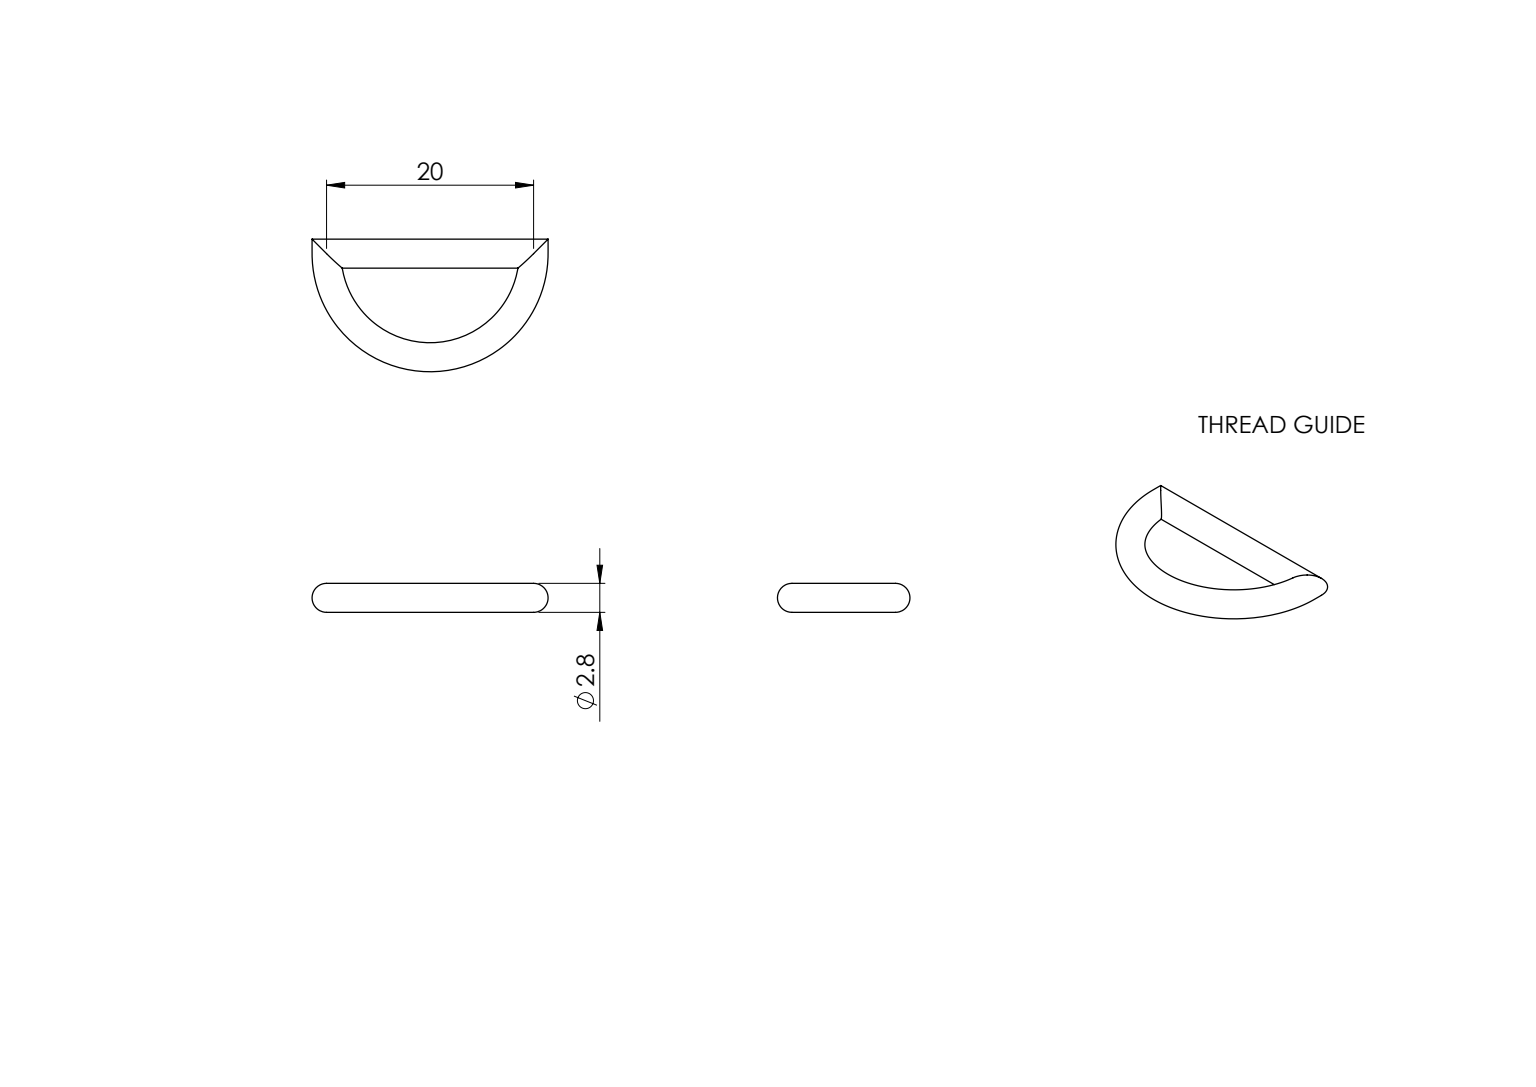
ISO-10303-21;
HEADER;
FILE_DESCRIPTION (('STEP AP214'),
    '1' );
FILE_NAME ('thread guide.step',
    '2026-10-25T11:00:22',
    ( '' ),
    ( '' ),
    'SwSTEP 2.0',
    'SolidWorks 2026',
    '' );
FILE_SCHEMA (( 'AUTOMOTIVE_DESIGN' ));
ENDSEC;

DATA;
#1=CARTESIAN_POINT ( 'NONE',  ( -6.877134118866000456, -50.00000000000000000, 5.285102517561346858 ) ) ;
#2=CARTESIAN_POINT ( 'NONE',  ( 11.39999999999999680, -52.79999999999999716, -0.5466666666666269991 ) ) ;
#3=ORIENTED_EDGE ( 'NONE', *, *, #2173, .T. ) ;
#9=( BOUNDED_SURFACE ( )  B_SPLINE_SURFACE ( 3, 3, ( 
 ( #2907, #429, #2418, #2187, #1154, #2219, #2974, #1713, #2728, #2169, #3178, #2938, #2958, #2662, #1219, #461, #1468, #698, #2482, #1435, #1899, #2449, #446, #1450, #649, #2462, #2236, #1651, #919, #1916, #663, #189, #680, #1664, #2679, #1419, #2432, #1171 ),
 ( #1682, #1596, #593, #2589, #838, #2249, #321, #302, #69, #2812, #1788, #1838, #1822, #2342, #3004, #817, #221, #2743, #3255, #1078, #1549, #337, #2094, #1730, #1292, #477, #787, #726, #801, #2001, #1486, #2308, #35, #2797, #984, #1343, #1045, #2610 ),
 ( #1233, #3101, #969, #2498, #1313, #2829, #1806, #2077, #1985, #559, #540, #2056, #2554, #1328, #2847, #2358, #2989, #285, #3065, #1561, #2324, #2567, #52, #1064, #3081, #575, #1578, #884, #87, #2898, #388, #899, #2112, #1910, #2672, #2930, #2396, #671 ),
 ( #372, #1672, #2689, #855, #150, #2916, #657, #3139, #1613, #1892, #2377, #3120, #2426, #2628, #912, #1163, #1925, #1131, #122, #2145, #1855, #3152, #2131, #1097, #2866, #2181, #1412, #643, #872, #608, #3185, #1629, #1644, #1873, #420, #2411, #1428, #1658 ),
 ( #355, #3169, #107, #2882, #627, #1362, #1116, #402, #2642, #1381, #2658, #1395, #134, #1145, #2162, #438, #2194, #736, #994, #1194, #961, #487, #1496, #2504, #1179, #2257, #705, #3234, #2210, #2763, #1476, #228, #1993, #453, #2492, #1444, #214, #1227 ),
 ( #1241, #167, #2751, #2011, #3265, #2456, #720, #499, #182, #2736, #3213, #3199, #1741, #3013, #943, #1978, #752, #1753, #2441, #2243, #1691, #927, #1961, #1941, #2967, #2949, #688, #2707, #2722, #1705, #1458, #2474, #2228, #198, #1210, #2981, #1722, #470 ),
 ( #3249, #975, #2998, #813, #765, #315, #1507, #1256, #797, #1307, #2303, #2564, #2519, #31, #1, #1784, #1768, #1817, #2823, #571, #1574, #1011, #2026, #1544, #2808, #2271, #830, #1323, #2582, #1801, #2338, #1039, #246, #2052, #554, #2319, #3026, #48 ) ),
 .UNSPECIFIED., .T., .F., .F. ) 
 B_SPLINE_SURFACE_WITH_KNOTS ( ( 4, 3, 4 ),
 ( 4, 2, 2, 2, 2, 2, 2, 2, 2, 2, 2, 2, 2, 2, 2, 2, 2, 2, 4 ),
 ( 0.000000000000000000, 0.5000000000000000000, 1.000000000000000000 ),
 ( -0.05205660780589810299, -0.02602830390294905150, 0.000000000000000000, 0.01562500000000000000, 0.03125000000000000000, 0.06250000000000000000, 0.1250000000000000000, 0.2500000000000000000, 0.3750000000000000000, 0.5000000000000000000, 0.6250000000000000000, 0.7500000000000000000, 0.8750000000000000000, 0.9375000000000000000, 0.9687500000000000000, 0.9843750000000000000, 1.000000000000000000, 1.026028303902949190, 1.052056607805898381 ),
 .UNSPECIFIED. ) 
 GEOMETRIC_REPRESENTATION_ITEM ( )  RATIONAL_B_SPLINE_SURFACE ( (
 ( 1.000000000000000000, 1.000000000000000000, 1.000000000000000000, 1.000000000000000000, 1.000000000000000000, 1.000000000000000000, 1.000000000000000000, 1.000000000000000000, 1.000000000000000000, 1.000000000000000000, 1.000000000000000000, 1.000000000000000000, 1.000000000000000000, 1.000000000000000000, 1.000000000000000000, 1.000000000000000000, 1.000000000000000000, 1.000000000000000000, 1.000000000000000000, 1.000000000000000000, 1.000000000000000000, 1.000000000000000000, 1.000000000000000000, 1.000000000000000000, 1.000000000000000000, 1.000000000000000000, 1.000000000000000000, 1.000000000000000000, 1.000000000000000000, 1.000000000000000000, 1.000000000000000000, 1.000000000000000000, 1.000000000000000000, 1.000000000000000000, 1.000000000000000000, 1.000000000000000000, 1.000000000000000000, 1.000000000000000000),
 ( 0.3333333333333333703, 0.3333333333333333703, 0.3333333333333333703, 0.3333333333333333703, 0.3333333333333333703, 0.3333333333333333703, 0.3333333333333333703, 0.3333333333333333703, 0.3333333333333333703, 0.3333333333333333703, 0.3333333333333333703, 0.3333333333333333703, 0.3333333333333333703, 0.3333333333333333703, 0.3333333333333333703, 0.3333333333333333703, 0.3333333333333333703, 0.3333333333333333703, 0.3333333333333333703, 0.3333333333333333703, 0.3333333333333333703, 0.3333333333333333703, 0.3333333333333333703, 0.3333333333333333703, 0.3333333333333333703, 0.3333333333333333703, 0.3333333333333333703, 0.3333333333333333703, 0.3333333333333333703, 0.3333333333333333703, 0.3333333333333333703, 0.3333333333333333703, 0.3333333333333333703, 0.3333333333333333703, 0.3333333333333333703, 0.3333333333333333703, 0.3333333333333333703, 0.3333333333333333703),
 ( 0.3333333333333333703, 0.3333333333333333703, 0.3333333333333333703, 0.3333333333333333703, 0.3333333333333333703, 0.3333333333333333703, 0.3333333333333333703, 0.3333333333333333703, 0.3333333333333333703, 0.3333333333333333703, 0.3333333333333333703, 0.3333333333333333703, 0.3333333333333333703, 0.3333333333333333703, 0.3333333333333333703, 0.3333333333333333703, 0.3333333333333333703, 0.3333333333333333703, 0.3333333333333333703, 0.3333333333333333703, 0.3333333333333333703, 0.3333333333333333703, 0.3333333333333333703, 0.3333333333333333703, 0.3333333333333333703, 0.3333333333333333703, 0.3333333333333333703, 0.3333333333333333703, 0.3333333333333333703, 0.3333333333333333703, 0.3333333333333333703, 0.3333333333333333703, 0.3333333333333333703, 0.3333333333333333703, 0.3333333333333333703, 0.3333333333333333703, 0.3333333333333333703, 0.3333333333333333703),
 ( 1.000000000000000000, 1.000000000000000000, 1.000000000000000000, 1.000000000000000000, 1.000000000000000000, 1.000000000000000000, 1.000000000000000000, 1.000000000000000000, 1.000000000000000000, 1.000000000000000000, 1.000000000000000000, 1.000000000000000000, 1.000000000000000000, 1.000000000000000000, 1.000000000000000000, 1.000000000000000000, 1.000000000000000000, 1.000000000000000000, 1.000000000000000000, 1.000000000000000000, 1.000000000000000000, 1.000000000000000000, 1.000000000000000000, 1.000000000000000000, 1.000000000000000000, 1.000000000000000000, 1.000000000000000000, 1.000000000000000000, 1.000000000000000000, 1.000000000000000000, 1.000000000000000000, 1.000000000000000000, 1.000000000000000000, 1.000000000000000000, 1.000000000000000000, 1.000000000000000000, 1.000000000000000000, 1.000000000000000000),
 ( 0.3333333333333333703, 0.3333333333333333703, 0.3333333333333333703, 0.3333333333333333703, 0.3333333333333333703, 0.3333333333333333703, 0.3333333333333333703, 0.3333333333333333703, 0.3333333333333333703, 0.3333333333333333703, 0.3333333333333333703, 0.3333333333333333703, 0.3333333333333333703, 0.3333333333333333703, 0.3333333333333333703, 0.3333333333333333703, 0.3333333333333333703, 0.3333333333333333703, 0.3333333333333333703, 0.3333333333333333703, 0.3333333333333333703, 0.3333333333333333703, 0.3333333333333333703, 0.3333333333333333703, 0.3333333333333333703, 0.3333333333333333703, 0.3333333333333333703, 0.3333333333333333703, 0.3333333333333333703, 0.3333333333333333703, 0.3333333333333333703, 0.3333333333333333703, 0.3333333333333333703, 0.3333333333333333703, 0.3333333333333333703, 0.3333333333333333703, 0.3333333333333333703, 0.3333333333333333703),
 ( 0.3333333333333333703, 0.3333333333333333703, 0.3333333333333333703, 0.3333333333333333703, 0.3333333333333333703, 0.3333333333333333703, 0.3333333333333333703, 0.3333333333333333703, 0.3333333333333333703, 0.3333333333333333703, 0.3333333333333333703, 0.3333333333333333703, 0.3333333333333333703, 0.3333333333333333703, 0.3333333333333333703, 0.3333333333333333703, 0.3333333333333333703, 0.3333333333333333703, 0.3333333333333333703, 0.3333333333333333703, 0.3333333333333333703, 0.3333333333333333703, 0.3333333333333333703, 0.3333333333333333703, 0.3333333333333333703, 0.3333333333333333703, 0.3333333333333333703, 0.3333333333333333703, 0.3333333333333333703, 0.3333333333333333703, 0.3333333333333333703, 0.3333333333333333703, 0.3333333333333333703, 0.3333333333333333703, 0.3333333333333333703, 0.3333333333333333703, 0.3333333333333333703, 0.3333333333333333703),
 ( 1.000000000000000000, 1.000000000000000000, 1.000000000000000000, 1.000000000000000000, 1.000000000000000000, 1.000000000000000000, 1.000000000000000000, 1.000000000000000000, 1.000000000000000000, 1.000000000000000000, 1.000000000000000000, 1.000000000000000000, 1.000000000000000000, 1.000000000000000000, 1.000000000000000000, 1.000000000000000000, 1.000000000000000000, 1.000000000000000000, 1.000000000000000000, 1.000000000000000000, 1.000000000000000000, 1.000000000000000000, 1.000000000000000000, 1.000000000000000000, 1.000000000000000000, 1.000000000000000000, 1.000000000000000000, 1.000000000000000000, 1.000000000000000000, 1.000000000000000000, 1.000000000000000000, 1.000000000000000000, 1.000000000000000000, 1.000000000000000000, 1.000000000000000000, 1.000000000000000000, 1.000000000000000000, 1.000000000000000000) ) ) 
 REPRESENTATION_ITEM ( '' )  SURFACE ( )  );
#12=CARTESIAN_POINT ( 'NONE',  ( 8.609154349733209699, -50.54332563323345795, 1.294262817214646644 ) ) ;
#13=CARTESIAN_POINT ( 'NONE',  ( -8.530791689320901483, -50.00000000000000000, 1.124695299888049504 ) ) ;
#15=EDGE_CURVE ( 'NONE', #50, #1696, #42, .T. ) ;
#28=CARTESIAN_POINT ( 'NONE',  ( 7.513445500750180805, -50.00000000000000000, 4.333070140107198043 ) ) ;
#31=CARTESIAN_POINT ( 'NONE',  ( -7.513445500749800665, -50.00000000000000000, 4.333070140105378165 ) ) ;
#35=CARTESIAN_POINT ( 'NONE',  ( 8.599996472200352571, -47.20000000000001705, 0.1525981975067867147 ) ) ;
#40=PRODUCT_DEFINITION_CONTEXT ( 'detailed design', #391, 'design' ) ;
#42=B_SPLINE_CURVE_WITH_KNOTS ( 'NONE', 3,
 ( #682, #3227, #1437, #2189, #1490, #1684, #3257, #223, #987, #191, #2464, #1205, #3193, #956 ),
 .UNSPECIFIED., .F., .F.,
 ( 4, 2, 2, 2, 2, 2, 4 ),
 ( -7.483321455827298351E-06, 0.0006606241027954298925, 0.001328731527046687205, 0.001662785239172322529, 0.001996838951297958287, 0.002330892663423593178, 0.002664946375549228936 ),
 .UNSPECIFIED. ) ;
#44=CARTESIAN_POINT ( 'NONE',  ( 8.599996472200352571, -50.00000000000000000, 0.1525981975067866592 ) ) ;
#48=CARTESIAN_POINT ( 'NONE',  ( 8.599999999999996092, -50.00000000000000000, -1.639999999999997460 ) ) ;
#50=VERTEX_POINT ( 'NONE', #715 ) ;
#52=CARTESIAN_POINT ( 'NONE',  ( 7.005833569766282132, -47.20000000000001705, 9.116201041261453142 ) ) ;
#61=CARTESIAN_POINT ( 'NONE',  ( 1.125736483476999839, -50.00000000000000000, 8.599999999999996092 ) ) ;
#66=CARTESIAN_POINT ( 'NONE',  ( -9.999999999999998224, -48.60000000000000142, 1.734719587726169024E-19 ) ) ;
#69=CARTESIAN_POINT ( 'NONE',  ( -8.572276570256935457, -47.20000000000001705, 0.7042094815226510596 ) ) ;
#77=CARTESIAN_POINT ( 'NONE',  ( -4.331939449206426929, -50.00000000000000000, 7.514224851276241957 ) ) ;
#83=CARTESIAN_POINT ( 'NONE',  ( 7.513445500750180805, -50.00000000000000000, 4.333070140107198043 ) ) ;
#87=CARTESIAN_POINT ( 'NONE',  ( 11.30825875096014066, -47.20000000000001705, 1.490875164968454625 ) ) ;
#91=CARTESIAN_POINT ( 'NONE',  ( -2.250215587473127332, -50.00000000000000000, 8.376503107917878665 ) ) ;
#93=VECTOR ( 'NONE', #127, 1000.000000000000000 ) ;
#107=CARTESIAN_POINT ( 'NONE',  ( -11.39999999999999680, -52.79999999999999716, -1.093333333333363022 ) ) ;
#109=FACE_OUTER_BOUND ( 'NONE', #857, .T. ) ;
#114=CARTESIAN_POINT ( 'NONE',  ( 8.599999999999996092, -50.00000000000000000, -0.5466666666666269991 ) ) ;
#117=SHAPE_REPRESENTATION_RELATIONSHIP ( 'NONE' , 'NONE' ,  #2799, #1401 ) ;
#119=CARTESIAN_POINT ( 'NONE',  ( -1.492255338562904265, -47.20000000000001705, 11.39999999999999680 ) ) ;
#122=CARTESIAN_POINT ( 'NONE',  ( -1.492255338562904043, -50.00000000000000000, 11.39999999999999680 ) ) ;
#127=DIRECTION ( 'NONE',  ( -1.000000000000000000, -0.000000000000000000, -0.000000000000000000 ) ) ;
#131=CARTESIAN_POINT ( 'NONE',  ( 11.39999999999999680, -47.20000000000001705, -0.5466666666666269991 ) ) ;
#134=CARTESIAN_POINT ( 'NONE',  ( -10.81682914263834405, -52.79999999999999716, 3.675996170188739143 ) ) ;
#137=CARTESIAN_POINT ( 'NONE',  ( -8.767617449782825645, -49.18583174968846805, 1.157007882117286446 ) ) ;
#139=ORIENTED_EDGE ( 'NONE', *, *, #3025, .T. ) ;
#141=CLOSED_SHELL ( 'NONE', ( #340, #1948, #3100, #1050 ) ) ;
#147=CARTESIAN_POINT ( 'NONE',  ( 11.03470001049147697, -47.20000000000001705, 2.958453039086267111 ) ) ;
#149=CARTESIAN_POINT ( 'NONE',  ( -10.97094949647943274, -51.01251636945237777, -0.9709494964794268546 ) ) ;
#150=CARTESIAN_POINT ( 'NONE',  ( -11.40000778997679021, -50.00000000000000000, -0.2924664341913127408 ) ) ;
#159=CARTESIAN_POINT ( 'NONE',  ( 9.354236102686614984, -48.73731279115568071, 0.6262106814100325547 ) ) ;
#163=CARTESIAN_POINT ( 'NONE',  ( -10.81682914263834405, -50.00000000000000000, 3.675996170188739143 ) ) ;
#164=CARTESIAN_POINT ( 'NONE',  ( -11.39999532361432522, -50.00000000000000000, 0.1755699507458657049 ) ) ;
#167=CARTESIAN_POINT ( 'NONE',  ( -8.599999999999996092, -52.79999999999999716, -1.366666666666159546 ) ) ;
#169=CARTESIAN_POINT ( 'NONE',  ( -8.582665138674013150, -50.00000000000000000, 0.5636706063486749407 ) ) ;
#174=B_SPLINE_CURVE_WITH_KNOTS ( 'NONE', 3,
 ( #727, #1234, #2700, #1436, #190, #493, #2002, #3005, #1747, #2526, #526, #1263 ),
 .UNSPECIFIED., .F., .F.,
 ( 4, 2, 2, 2, 2, 4 ),
 ( 0.002664946375549201180, 0.002999773306175300240, 0.003334600236801398866, 0.004004254098053579639, 0.004673907959305761278, 0.005343561820557941183 ),
 .UNSPECIFIED. ) ;
#179=CARTESIAN_POINT ( 'NONE',  ( -11.39539595717859299, -47.20000000000001705, 0.3739757293043587949 ) ) ;
#182=CARTESIAN_POINT ( 'NONE',  ( -8.572276570256935457, -52.79999999999999716, 0.7042094815226510596 ) ) ;
#184=CARTESIAN_POINT ( 'NONE',  ( -1.125736483476999839, -50.00000000000000000, 8.599999999999996092 ) ) ;
#186=CARTESIAN_POINT ( 'NONE',  ( 11.38641147205292725, -49.77694418854823510, -1.386411472052930804 ) ) ;
#189=CARTESIAN_POINT ( 'NONE',  ( 8.596526774713712626, -50.00000000000000000, 0.2821220414049827596 ) ) ;
#190=CARTESIAN_POINT ( 'NONE',  ( -11.29810924534245586, -49.46572717680115971, -1.298109245342457418 ) ) ;
#191=CARTESIAN_POINT ( 'NONE',  ( 11.29771452881883498, -50.53508261979053628, -1.297714528818850299 ) ) ;
#194=CARTESIAN_POINT ( 'NONE',  ( -11.40000778997679198, -52.79999999999999716, -0.2924664341913127408 ) ) ;
#198=CARTESIAN_POINT ( 'NONE',  ( 8.600005876649037262, -52.79999999999999716, -0.2541998246239300374 ) ) ;
#200=CARTESIAN_POINT ( 'NONE',  ( -8.572276570256935457, -50.00000000000000000, 0.7042094815226510596 ) ) ;
#202=CARTESIAN_POINT ( 'NONE',  ( 9.999999999999976907, -48.60000000000000142, -1.084199742356775455E-20 ) ) ;
#203=ORIENTED_EDGE ( 'NONE', *, *, #2410, .F. ) ;
#210=CARTESIAN_POINT ( 'NONE',  ( -9.959683570761574956, -52.79999999999999716, 5.743837162464267898 ) ) ;
#212=CARTESIAN_POINT ( 'NONE',  ( -11.39999999999999680, -50.11112248448768014, -1.400000000000000355 ) ) ;
#214=CARTESIAN_POINT ( 'NONE',  ( 11.39999999999999680, -52.79999999999999716, -1.366666666666861873 ) ) ;
#217=CARTESIAN_POINT ( 'NONE',  ( 6.877134118866902845, -50.00000000000000000, 5.285102517562147995 ) ) ;
#221=CARTESIAN_POINT ( 'NONE',  ( -4.331939449206426929, -47.20000000000001705, 7.514224851276242845 ) ) ;
#223=CARTESIAN_POINT ( 'NONE',  ( 11.15228598338264732, -50.80068377669682889, -1.152285983382657086 ) ) ;
#225=CARTESIAN_POINT ( 'NONE',  ( 11.39999999999999680, -50.00000000000000000, -1.093333333333372126 ) ) ;
#228=CARTESIAN_POINT ( 'NONE',  ( 11.39539595717845799, -52.79999999999999716, 0.3739757293042010877 ) ) ;
#231=CARTESIAN_POINT ( 'NONE',  ( -8.582665138674013150, -47.20000000000001705, 0.5636706063486748297 ) ) ;
#236=UNCERTAINTY_MEASURE_WITH_UNIT (LENGTH_MEASURE( 1.000000000000000082E-05 ), #1255, 'distance_accuracy_value', 'NONE');
#241=CARTESIAN_POINT ( 'NONE',  ( -1.492255338562904265, -52.79999999999999716, 11.39999999999999680 ) ) ;
#246=CARTESIAN_POINT ( 'NONE',  ( 8.599996472200352571, -50.00000000000000000, 0.1525981975067866592 ) ) ;
#258=CARTESIAN_POINT ( 'NONE',  ( -8.596526774713705521, -52.79999999999999716, 0.2821220414048196123 ) ) ;
#274=CARTESIAN_POINT ( 'NONE',  ( 8.564669657331105412, -50.44377267524160402, 1.332368788789859204 ) ) ;
#276=CARTESIAN_POINT ( 'NONE',  ( -8.599999999999996092, -50.00000000000000000, -0.5466666666666361030 ) ) ;
#285=CARTESIAN_POINT ( 'NONE',  ( -2.982843918280285944, -47.20000000000001705, 11.10373667793902541 ) ) ;
#292=CARTESIAN_POINT ( 'NONE',  ( 9.199433601069458177, -51.18229052107441390, 0.7695943483561379361 ) ) ;
#293=CARTESIAN_POINT ( 'NONE',  ( 8.324422814932070480, -50.00000000000000000, 2.231815450537910639 ) ) ;
#302=CARTESIAN_POINT ( 'NONE',  ( -8.582665138674013150, -47.20000000000001705, 0.5636706063486748297 ) ) ;
#306=EDGE_CURVE ( 'NONE', #661, #403, #2966, .T. ) ;
#311=CARTESIAN_POINT ( 'NONE',  ( -5.285102517542626721, -50.00000000000000000, 6.877134118847252786 ) ) ;
#315=CARTESIAN_POINT ( 'NONE',  ( -8.599996472200352571, -50.00000000000000000, 0.1525981975067654262 ) ) ;
#321=CARTESIAN_POINT ( 'NONE',  ( -8.596526774713705521, -47.20000000000001705, 0.2821220414048196123 ) ) ;
#329=CARTESIAN_POINT ( 'NONE',  ( 8.599999999999996092, -52.79999999999999716, -1.093333333333372126 ) ) ;
#337=CARTESIAN_POINT ( 'NONE',  ( 4.331939449206418047, -47.20000000000001705, 7.514224851275111305 ) ) ;
#340=ADVANCED_FACE ( 'NONE', ( #832 ), #2291, .T. ) ;
#341=CARTESIAN_POINT ( 'NONE',  ( -5.285102517542626721, -50.00000000000000000, 6.877134118847252786 ) ) ;
#345=CARTESIAN_POINT ( 'NONE',  ( 9.676554491074602637, -48.63437908886126593, 0.3185635799549096925 ) ) ;
#355=CARTESIAN_POINT ( 'NONE',  ( -11.39999999999999680, -52.79999999999999716, -1.639999999999997460 ) ) ;
#365=VERTEX_POINT ( 'NONE', #66 ) ;
#368=CARTESIAN_POINT ( 'NONE',  ( -9.959683570761574956, -47.20000000000001705, 5.743837162464267898 ) ) ;
#369=CARTESIAN_POINT ( 'NONE',  ( -11.39999999999999680, -50.00000000000000000, -1.400000000000000133 ) ) ;
#372=CARTESIAN_POINT ( 'NONE',  ( -11.39999999999999680, -50.00000000000000000, -1.639999999999997460 ) ) ;
#379=CARTESIAN_POINT ( 'NONE',  ( 8.485280282859413603, -50.00000000000000000, 1.400000000000001021 ) ) ;
#381=CARTESIAN_POINT ( 'NONE',  ( 11.39999999999999680, -50.00000000000000000, -1.400000000003877254 ) ) ;
#382=( LENGTH_UNIT ( ) NAMED_UNIT ( * ) SI_UNIT ( .MILLI., .METRE. ) );
#383=CARTESIAN_POINT ( 'NONE',  ( -11.30825875096001454, -50.00000000000000000, 1.490875164968288757 ) ) ;
#388=CARTESIAN_POINT ( 'NONE',  ( 11.37702123033534995, -47.20000000000001705, 0.7471912688806705560 ) ) ;
#391=APPLICATION_CONTEXT ( 'automotive_design' ) ;
#398=CARTESIAN_POINT ( 'NONE',  ( -11.25335008359214584, -47.20000000000001705, 1.860476840075229843 ) ) ;
#399=CARTESIAN_POINT ( 'NONE',  ( -9.116201041288242379, -50.00000000000000000, 7.005833569791151128 ) ) ;
#402=CARTESIAN_POINT ( 'NONE',  ( -11.37702123033521850, -52.79999999999999716, 0.7471912688805021352 ) ) ;
#403=VERTEX_POINT ( 'NONE', #2824 ) ;
#417=CARTESIAN_POINT ( 'NONE',  ( -11.25335008359228794, -50.00000000000000000, 1.860476840075229621 ) ) ;
#420=CARTESIAN_POINT ( 'NONE',  ( 11.39999999999999680, -50.00000000000000000, -0.5466666666666269991 ) ) ;
#423=CARTESIAN_POINT ( 'NONE',  ( -2.250215587473127332, -50.00000000000000000, 8.376503107917878665 ) ) ;
#429=CARTESIAN_POINT ( 'NONE',  ( -8.599999999999996092, -50.00000000000000000, -1.366666666666159768 ) ) ;
#435=CARTESIAN_POINT ( 'NONE',  ( -11.39999532361432522, -47.20000000000001705, 0.1755699507458657049 ) ) ;
#436=CARTESIAN_POINT ( 'NONE',  ( -2.982843918280285944, -50.00000000000000000, 11.10373667793902541 ) ) ;
#438=CARTESIAN_POINT ( 'NONE',  ( -7.005833569766191538, -52.79999999999999716, 9.116201041262108618 ) ) ;
#440=CARTESIAN_POINT ( 'NONE',  ( -8.324422814933019055, -50.00000000000000000, 2.231815450536601464 ) ) ;
#446=CARTESIAN_POINT ( 'NONE',  ( 5.285102517541700351, -50.00000000000000000, 6.877134118846478295 ) ) ;
#450=CARTESIAN_POINT ( 'NONE',  ( 11.36325033731725576, -52.79999999999999716, 0.9334869871343942638 ) ) ;
#451=CARTESIAN_POINT ( 'NONE',  ( 11.39999999999999680, -50.00000000000000000, -1.013333333334534458 ) ) ;
#452=CARTESIAN_POINT ( 'NONE',  ( -11.38628138490143371, -50.22360298513551413, -1.386281384901433045 ) ) ;
#453=CARTESIAN_POINT ( 'NONE',  ( 11.40000778997679198, -52.79999999999999716, -0.2924664341912773247 ) ) ;
#455=CARTESIAN_POINT ( 'NONE',  ( -8.600005876649037262, -47.20000000000001705, -0.2541998246238979520 ) ) ;
#460=( GEOMETRIC_REPRESENTATION_CONTEXT ( 3 ) GLOBAL_UNCERTAINTY_ASSIGNED_CONTEXT ( ( #236 ) ) GLOBAL_UNIT_ASSIGNED_CONTEXT ( ( #1255, #1270, #3012 ) ) REPRESENTATION_CONTEXT ( 'NONE', 'WORKASPACE' ) );
#461=CARTESIAN_POINT ( 'NONE',  ( -5.285102517542626721, -50.00000000000000000, 6.877134118847252786 ) ) ;
#467=CARTESIAN_POINT ( 'NONE',  ( 11.39539595717853082, -50.00000000000000000, 0.3739757293042009212 ) ) ;
#470=CARTESIAN_POINT ( 'NONE',  ( 8.599999999999996092, -52.79999999999999716, -1.639999999999997460 ) ) ;
#472=CARTESIAN_POINT ( 'NONE',  ( -1.125736483477000061, -47.20000000000001705, 8.599999999999996092 ) ) ;
#474=CARTESIAN_POINT ( 'NONE',  ( 10.15784101500072190, -48.59999999999998010, -0.1578371243778893540 ) ) ;
#477=CARTESIAN_POINT ( 'NONE',  ( 8.160064090060387798, -47.20000000000001705, 2.773119917860402239 ) ) ;
#481=CARTESIAN_POINT ( 'NONE',  ( 9.838268070989578007, -51.39301687163384003, 0.1607570464466796800 ) ) ;
#483=CARTESIAN_POINT ( 'NONE',  ( -7.005833569766191538, -52.79999999999999716, 9.116201041262108618 ) ) ;
#484=CARTESIAN_POINT ( 'NONE',  ( 11.25335008359272493, -50.00000000000000000, 1.860476840074170246 ) ) ;
#487=CARTESIAN_POINT ( 'NONE',  ( 5.742338339644331491, -52.79999999999999716, 9.960716663318304853 ) ) ;
#489=CARTESIAN_POINT ( 'NONE',  ( 2.250215587473118450, -47.20000000000001705, 8.376503107919017310 ) ) ;
#493=CARTESIAN_POINT ( 'NONE',  ( -11.16040725319408011, -49.19031162998081186, -1.160407253194084332 ) ) ;
#496=CARTESIAN_POINT ( 'NONE',  ( 10.81682914263883610, -50.00000000000000000, 3.675996170187548540 ) ) ;
#499=CARTESIAN_POINT ( 'NONE',  ( -8.582665138674013150, -52.79999999999999716, 0.5636706063486748297 ) ) ;
#507=EDGE_CURVE ( 'NONE', #890, #1696, #1738, .T. ) ;
#513=CARTESIAN_POINT ( 'NONE',  ( -8.599999999999996092, -52.79999999999999716, -1.093333333333363022 ) ) ;
#514=ORIENTED_EDGE ( 'NONE', *, *, #1474, .T. ) ;
#526=CARTESIAN_POINT ( 'NONE',  ( -10.15784101513766835, -48.60000000000000853, -0.1578371242409689901 ) ) ;
#530=CARTESIAN_POINT ( 'NONE',  ( 9.999999999999989342, -51.39999999999999147, -1.084199742081416524E-20 ) ) ;
#531=CARTESIAN_POINT ( 'NONE',  ( 8.530791689320604831, -50.00000000000000000, 1.124695299888175182 ) ) ;
#540=CARTESIAN_POINT ( 'NONE',  ( -11.25335008359214584, -47.20000000000001705, 1.860476840075229843 ) ) ;
#549=CARTESIAN_POINT ( 'NONE',  ( -8.324422814933019055, -52.79999999999999716, 2.231815450536601020 ) ) ;
#554=CARTESIAN_POINT ( 'NONE',  ( 8.599999999999996092, -50.00000000000000000, -0.5466666666666269991 ) ) ;
#556=ORIENTED_EDGE ( 'NONE', *, *, #2233, .T. ) ;
#559=CARTESIAN_POINT ( 'NONE',  ( -11.30825875096015665, -47.20000000000001705, 1.490875164968288979 ) ) ;
#566=CARTESIAN_POINT ( 'NONE',  ( 8.599999999999996092, -52.79999999999999716, -0.5466666666666269991 ) ) ;
#571=CARTESIAN_POINT ( 'NONE',  ( 1.125736483476999839, -50.00000000000000000, 8.599999999999996092 ) ) ;
#575=CARTESIAN_POINT ( 'NONE',  ( 10.81682914263912210, -47.20000000000001705, 3.675996170187548540 ) ) ;
#581=CARTESIAN_POINT ( 'NONE',  ( 8.600005876649037262, -52.79999999999999716, -0.2541998246239300374 ) ) ;
#593=CARTESIAN_POINT ( 'NONE',  ( -8.599999999999996092, -47.20000000000001705, -1.093333333333363022 ) ) ;
#594=PRODUCT_DEFINITION_FORMATION_WITH_SPECIFIED_SOURCE ( 'ANY', '', #654, .NOT_KNOWN. ) ;
#600=CARTESIAN_POINT ( 'NONE',  ( 8.160064090060387798, -50.00000000000000000, 2.773119917860402239 ) ) ;
#608=CARTESIAN_POINT ( 'NONE',  ( 11.36325033731732503, -50.00000000000000000, 0.9334869871343942638 ) ) ;
#610=CARTESIAN_POINT ( 'NONE',  ( -9.920079092145705602, -48.60000000000000142, 0.07989781697764072876 ) ) ;
#620=FILL_AREA_STYLE_COLOUR ( '', #2179 ) ;
#622=CARTESIAN_POINT ( 'NONE',  ( 8.599996472200352571, -47.20000000000001705, 0.1525981975067867147 ) ) ;
#627=CARTESIAN_POINT ( 'NONE',  ( -11.40000778997679198, -52.79999999999999716, -0.2924664341913127408 ) ) ;
#629=CARTESIAN_POINT ( 'NONE',  ( -9.354236102686607879, -48.73731279115566650, 0.6262106814100150132 ) ) ;
#639=CARTESIAN_POINT ( 'NONE',  ( 11.36325033731739609, -47.20000000000001705, 0.9334869871343942638 ) ) ;
#643=CARTESIAN_POINT ( 'NONE',  ( 11.25335008359272493, -50.00000000000000000, 1.860476840074170246 ) ) ;
#649=CARTESIAN_POINT ( 'NONE',  ( 7.513445500750180805, -50.00000000000000000, 4.333070140107198043 ) ) ;
#653=CARTESIAN_POINT ( 'NONE',  ( -11.40000778997679021, -50.00000000000000000, -0.2924664341913127408 ) ) ;
#654=PRODUCT ( 'thread guide', 'thread guide', '', ( #1244 ) ) ;
#657=CARTESIAN_POINT ( 'NONE',  ( -11.39539595717866405, -50.00000000000000000, 0.3739757293043588504 ) ) ;
#660=CARTESIAN_POINT ( 'NONE',  ( -9.838139443699130737, -48.60697500979578933, 0.1608869294866560606 ) ) ;
#661=VERTEX_POINT ( 'NONE', #3071 ) ;
#663=CARTESIAN_POINT ( 'NONE',  ( 8.582665138674004268, -50.00000000000000000, 0.5636706063485154017 ) ) ;
#667=CARTESIAN_POINT ( 'NONE',  ( 11.39539595717860188, -47.20000000000001705, 0.3739757293042009767 ) ) ;
#671=CARTESIAN_POINT ( 'NONE',  ( 11.39999999999999680, -47.20000000000001705, -1.639999999999997460 ) ) ;
#674=CARTESIAN_POINT ( 'NONE',  ( 8.572276570257082895, -47.20000000000001705, 0.7042094815225934390 ) ) ;
#680=CARTESIAN_POINT ( 'NONE',  ( 8.599996472200352571, -50.00000000000000000, 0.1525981975067866592 ) ) ;
#681=CARTESIAN_POINT ( 'NONE',  ( 9.838139443699079223, -48.60697500979577512, 0.1608869294865812039 ) ) ;
#682=CARTESIAN_POINT ( 'NONE',  ( 9.999999999999989342, -51.39999999999999147, -1.084199742081416524E-20 ) ) ;
#685=CARTESIAN_POINT ( 'NONE',  ( 9.116201041286979390, -47.20000000000001705, 7.005833569791843907 ) ) ;
#686=CARTESIAN_POINT ( 'NONE',  ( 11.39539595717853082, -50.00000000000000000, 0.3739757293042009212 ) ) ;
#687=CARTESIAN_POINT ( 'NONE',  ( -9.358389811592287444, -51.26439022220001362, 0.6222967749777322810 ) ) ;
#688=CARTESIAN_POINT ( 'NONE',  ( 8.324422814932072257, -52.79999999999999716, 2.231815450537910195 ) ) ;
#691=CARTESIAN_POINT ( 'NONE',  ( -7.513445500749800665, -50.00000000000000000, 4.333070140105378165 ) ) ;
#697=EDGE_CURVE ( 'NONE', #50, #403, #3126, .T. ) ;
#698=CARTESIAN_POINT ( 'NONE',  ( -2.250215587473127332, -50.00000000000000000, 8.376503107917878665 ) ) ;
#702=CARTESIAN_POINT ( 'NONE',  ( -10.81682914263834405, -52.79999999999999716, 3.675996170188739143 ) ) ;
#704=CARTESIAN_POINT ( 'NONE',  ( -9.838268070989617087, -51.39301687163386134, 0.1607570464467989457 ) ) ;
#705=CARTESIAN_POINT ( 'NONE',  ( 11.03470001049091032, -52.79999999999999716, 2.958453039085699565 ) ) ;
#707=CARTESIAN_POINT ( 'NONE',  ( 2.250215587473118450, -50.00000000000000000, 8.376503107919017310 ) ) ;
#715=CARTESIAN_POINT ( 'NONE',  ( 9.999999999999989342, -51.39999999999999147, -1.084199742081416524E-20 ) ) ;
#717=CARTESIAN_POINT ( 'NONE',  ( 11.30825875096028099, -50.00000000000000000, 1.490875164968454181 ) ) ;
#720=CARTESIAN_POINT ( 'NONE',  ( -8.596526774713705521, -52.79999999999999716, 0.2821220414048196123 ) ) ;
#722=CARTESIAN_POINT ( 'NONE',  ( -7.513445500749801553, -47.20000000000001705, 4.333070140105379942 ) ) ;
#724=CARTESIAN_POINT ( 'NONE',  ( 11.40000000000000036, -49.88862030549577042, -1.399999999999994360 ) ) ;
#726=CARTESIAN_POINT ( 'NONE',  ( 8.489369361306732031, -47.20000000000001705, 1.403517616196621409 ) ) ;
#727=CARTESIAN_POINT ( 'NONE',  ( -11.39999999999999680, -50.00000000000000000, -1.400000000000000133 ) ) ;
#730=CARTESIAN_POINT ( 'NONE',  ( -8.599999999999996092, -50.00000000000000000, -0.5466666666666361030 ) ) ;
#733=CARTESIAN_POINT ( 'NONE',  ( 10.81682914263855544, -52.79999999999999716, 3.675996170187548540 ) ) ;
#736=CARTESIAN_POINT ( 'NONE',  ( -2.982843918280285944, -52.79999999999999716, 11.10373667793902541 ) ) ;
#738=CARTESIAN_POINT ( 'NONE',  ( -2.250215587473127332, -47.20000000000001705, 8.376503107917878665 ) ) ;
#749=CARTESIAN_POINT ( 'NONE',  ( 11.39999999999999680, -52.79999999999999716, -1.639999999999997460 ) ) ;
#750=CARTESIAN_POINT ( 'NONE',  ( 11.03470001049119453, -50.00000000000000000, 2.958453039085983338 ) ) ;
#752=CARTESIAN_POINT ( 'NONE',  ( -4.331939449206426929, -52.79999999999999716, 7.514224851276242845 ) ) ;
#762=CARTESIAN_POINT ( 'NONE',  ( 1.492255338562904043, -50.00000000000000000, 11.39999999999999680 ) ) ;
#765=CARTESIAN_POINT ( 'NONE',  ( -8.600005876649037262, -50.00000000000000000, -0.2541998246238979520 ) ) ;
#777=CARTESIAN_POINT ( 'NONE',  ( 9.358389811594321372, -51.26439022220082364, 0.6222967749758763212 ) ) ;
#778=CARTESIAN_POINT ( 'NONE',  ( -2.250215587473127332, -52.79999999999999716, 8.376503107917878665 ) ) ;
#787=CARTESIAN_POINT ( 'NONE',  ( 8.324422814932072257, -47.20000000000001705, 2.231815450537910195 ) ) ;
#793=CARTESIAN_POINT ( 'NONE',  ( -8.600005876649037262, -50.00000000000000000, -0.2541998246238979520 ) ) ;
#797=CARTESIAN_POINT ( 'NONE',  ( -8.572276570256935457, -50.00000000000000000, 0.7042094815226510596 ) ) ;
#798=CARTESIAN_POINT ( 'NONE',  ( 11.64000000000000057, -50.00000000000000000, 0.000000000000000000 ) ) ;
#801=CARTESIAN_POINT ( 'NONE',  ( 8.530791689320606608, -47.20000000000001705, 1.124695299888175182 ) ) ;
#809=CARTESIAN_POINT ( 'NONE',  ( -8.489369361306263073, -52.79999999999999716, 1.403517616197273554 ) ) ;
#813=CARTESIAN_POINT ( 'NONE',  ( -8.599999999999996092, -50.00000000000000000, -0.5466666666666361030 ) ) ;
#817=CARTESIAN_POINT ( 'NONE',  ( -5.285102517542626721, -47.20000000000001705, 6.877134118847253674 ) ) ;
#824=CARTESIAN_POINT ( 'NONE',  ( 6.877134118866901957, -52.79999999999999716, 5.285102517562147995 ) ) ;
#830=CARTESIAN_POINT ( 'NONE',  ( 8.324422814932070480, -50.00000000000000000, 2.231815450537910639 ) ) ;
#832=FACE_OUTER_BOUND ( 'NONE', #1836, .T. ) ;
#838=CARTESIAN_POINT ( 'NONE',  ( -8.600005876649037262, -47.20000000000001705, -0.2541998246238979520 ) ) ;
#844=CARTESIAN_POINT ( 'NONE',  ( 8.572276570257082895, -52.79999999999999716, 0.7042094815225934390 ) ) ;
#855=CARTESIAN_POINT ( 'NONE',  ( -11.39999999999999680, -50.00000000000000000, -0.5466666666666361030 ) ) ;
#857=EDGE_LOOP ( 'NONE', ( #3078, #2844, #1367, #3, #1429, #1404 ) ) ;
#860=ORIENTED_EDGE ( 'NONE', *, *, #3025, .F. ) ;
#868=CARTESIAN_POINT ( 'NONE',  ( 11.39999999999999680, -47.20000000000001705, -1.366666666666861873 ) ) ;
#869=CARTESIAN_POINT ( 'NONE',  ( -11.40000778997679021, -50.00000000000000000, -0.2924664341913127408 ) ) ;
#872=CARTESIAN_POINT ( 'NONE',  ( 11.30825875096028099, -50.00000000000000000, 1.490875164968454181 ) ) ;
#880=( NAMED_UNIT ( * ) SI_UNIT ( $, .STERADIAN. ) SOLID_ANGLE_UNIT ( ) );
#881=CARTESIAN_POINT ( 'NONE',  ( -9.116201041289377471, -47.20000000000001705, 7.005833569791151128 ) ) ;
#884=CARTESIAN_POINT ( 'NONE',  ( 11.25335008359258282, -47.20000000000001705, 1.860476840074028360 ) ) ;
#885=ORIENTED_EDGE ( 'NONE', *, *, #2233, .F. ) ;
#889=EDGE_CURVE ( 'NONE', #1696, #890, #2872, .T. ) ;
#890=VERTEX_POINT ( 'NONE', #2577 ) ;
#895=CARTESIAN_POINT ( 'NONE',  ( 11.39999532361432522, -47.20000000000001705, 0.1755699507458462760 ) ) ;
#898=VECTOR ( 'NONE', #3020, 1000.000000000000000 ) ;
#899=CARTESIAN_POINT ( 'NONE',  ( 11.39539595717860188, -47.20000000000001705, 0.3739757293042009767 ) ) ;
#901=( BOUNDED_SURFACE ( )  B_SPLINE_SURFACE ( 3, 3, ( 
 ( #1734, #2746, #2992, #730, #1989, #2709, #2754, #169, #200, #3201, #1446, #440, #2495, #691, #1944, #2458, #1480, #423, #184, #1744, #707, #1213, #2230, #217, #1229, #1196, #977, #1707, #1980, #1694, #2214, #930, #2983, #3215, #946, #2951, #2196, #963 ),
 ( #2724, #1964, #2691, #2969, #455, #1460, #2477, #231, #3236, #2506, #2245, #1430, #2443, #722, #1243, #1724, #2739, #738, #472, #3251, #489, #2259, #1995, #3001, #1498, #1181, #914, #1927, #2932, #674, #1675, #3166, #622, #2453, #1937, #1176, #2423, #2943 ),
 ( #3183, #2878, #2668, #2407, #1686, #435, #179, #1625, #1407, #2639, #398, #910, #1158, #368, #881, #1668, #1640, #1377, #119, #2913, #1440, #2704, #1423, #685, #1127, #2438, #147, #2191, #1655, #639, #1191, #667, #895, #2176, #131, #3133, #868, #2685 ),
 ( #2654, #1869, #2393, #1392, #653, #2895, #2142, #1921, #3196, #383, #417, #2926, #163, #923, #3149, #1141, #1887, #2158, #1906, #762, #1454, #1492, #1207, #2733, #1719, #496, #1975, #3231, #717, #2760, #1702, #467, #3023, #1990, #2502, #225, #1505, #2516 ),
 ( #2993, #2978, #1472, #2223, #194, #2253, #972, #958, #2487, #3210, #2963, #1224, #702, #210, #3261, #483, #2240, #2719, #241, #2468, #1008, #2205, #1956, #1238, #2006, #733, #991, #939, #1735, #450, #3246, #2747, #1253, #2267, #2, #2023, #3009, #749 ),
 ( #1750, #1765, #513, #2773, #1521, #2529, #258, #3089, #1318, #1019, #809, #549, #3109, #1845, #1603, #3035, #2819, #778, #1813, #2334, #2578, #1780, #2301, #824, #3053, #2787, #1540, #1052, #2858, #844, #2837, #1086, #2548, #581, #566, #329, #3072, #2049 ),
 ( #2036, #2599, #2068, #276, #793, #1335, #2349, #1301, #1798, #13, #2100, #2804, #1568, #1035, #2619, #311, #77, #1555, #1830, #61, #1070, #2085, #1585, #2560, #28, #600, #293, #1268, #531, #2286, #1283, #2317, #44, #1917, #114, #1370, #2139, #906 ) ),
 .UNSPECIFIED., .T., .F., .T. ) 
 B_SPLINE_SURFACE_WITH_KNOTS ( ( 4, 3, 4 ),
 ( 4, 2, 2, 2, 2, 2, 2, 2, 2, 2, 2, 2, 2, 2, 2, 2, 2, 2, 4 ),
 ( 0.000000000000000000, 0.5000000000000000000, 1.000000000000000000 ),
 ( -0.05205660780589810299, -0.02602830390294905150, 0.000000000000000000, 0.01562500000000000000, 0.03125000000000000000, 0.06250000000000000000, 0.1250000000000000000, 0.2500000000000000000, 0.3750000000000000000, 0.5000000000000000000, 0.6250000000000000000, 0.7500000000000000000, 0.8750000000000000000, 0.9375000000000000000, 0.9687500000000000000, 0.9843750000000000000, 1.000000000000000000, 1.026028303902949190, 1.052056607805898381 ),
 .UNSPECIFIED. ) 
 GEOMETRIC_REPRESENTATION_ITEM ( )  RATIONAL_B_SPLINE_SURFACE ( (
 ( 1.000000000000000000, 1.000000000000000000, 1.000000000000000000, 1.000000000000000000, 1.000000000000000000, 1.000000000000000000, 1.000000000000000000, 1.000000000000000000, 1.000000000000000000, 1.000000000000000000, 1.000000000000000000, 1.000000000000000000, 1.000000000000000000, 1.000000000000000000, 1.000000000000000000, 1.000000000000000000, 1.000000000000000000, 1.000000000000000000, 1.000000000000000000, 1.000000000000000000, 1.000000000000000000, 1.000000000000000000, 1.000000000000000000, 1.000000000000000000, 1.000000000000000000, 1.000000000000000000, 1.000000000000000000, 1.000000000000000000, 1.000000000000000000, 1.000000000000000000, 1.000000000000000000, 1.000000000000000000, 1.000000000000000000, 1.000000000000000000, 1.000000000000000000, 1.000000000000000000, 1.000000000000000000, 1.000000000000000000),
 ( 0.3333333333333333703, 0.3333333333333333703, 0.3333333333333333703, 0.3333333333333333703, 0.3333333333333333703, 0.3333333333333333703, 0.3333333333333333703, 0.3333333333333333703, 0.3333333333333333703, 0.3333333333333333703, 0.3333333333333333703, 0.3333333333333333703, 0.3333333333333333703, 0.3333333333333333703, 0.3333333333333333703, 0.3333333333333333703, 0.3333333333333333703, 0.3333333333333333703, 0.3333333333333333703, 0.3333333333333333703, 0.3333333333333333703, 0.3333333333333333703, 0.3333333333333333703, 0.3333333333333333703, 0.3333333333333333703, 0.3333333333333333703, 0.3333333333333333703, 0.3333333333333333703, 0.3333333333333333703, 0.3333333333333333703, 0.3333333333333333703, 0.3333333333333333703, 0.3333333333333333703, 0.3333333333333333703, 0.3333333333333333703, 0.3333333333333333703, 0.3333333333333333703, 0.3333333333333333703),
 ( 0.3333333333333333703, 0.3333333333333333703, 0.3333333333333333703, 0.3333333333333333703, 0.3333333333333333703, 0.3333333333333333703, 0.3333333333333333703, 0.3333333333333333703, 0.3333333333333333703, 0.3333333333333333703, 0.3333333333333333703, 0.3333333333333333703, 0.3333333333333333703, 0.3333333333333333703, 0.3333333333333333703, 0.3333333333333333703, 0.3333333333333333703, 0.3333333333333333703, 0.3333333333333333703, 0.3333333333333333703, 0.3333333333333333703, 0.3333333333333333703, 0.3333333333333333703, 0.3333333333333333703, 0.3333333333333333703, 0.3333333333333333703, 0.3333333333333333703, 0.3333333333333333703, 0.3333333333333333703, 0.3333333333333333703, 0.3333333333333333703, 0.3333333333333333703, 0.3333333333333333703, 0.3333333333333333703, 0.3333333333333333703, 0.3333333333333333703, 0.3333333333333333703, 0.3333333333333333703),
 ( 1.000000000000000000, 1.000000000000000000, 1.000000000000000000, 1.000000000000000000, 1.000000000000000000, 1.000000000000000000, 1.000000000000000000, 1.000000000000000000, 1.000000000000000000, 1.000000000000000000, 1.000000000000000000, 1.000000000000000000, 1.000000000000000000, 1.000000000000000000, 1.000000000000000000, 1.000000000000000000, 1.000000000000000000, 1.000000000000000000, 1.000000000000000000, 1.000000000000000000, 1.000000000000000000, 1.000000000000000000, 1.000000000000000000, 1.000000000000000000, 1.000000000000000000, 1.000000000000000000, 1.000000000000000000, 1.000000000000000000, 1.000000000000000000, 1.000000000000000000, 1.000000000000000000, 1.000000000000000000, 1.000000000000000000, 1.000000000000000000, 1.000000000000000000, 1.000000000000000000, 1.000000000000000000, 1.000000000000000000),
 ( 0.3333333333333333703, 0.3333333333333333703, 0.3333333333333333703, 0.3333333333333333703, 0.3333333333333333703, 0.3333333333333333703, 0.3333333333333333703, 0.3333333333333333703, 0.3333333333333333703, 0.3333333333333333703, 0.3333333333333333703, 0.3333333333333333703, 0.3333333333333333703, 0.3333333333333333703, 0.3333333333333333703, 0.3333333333333333703, 0.3333333333333333703, 0.3333333333333333703, 0.3333333333333333703, 0.3333333333333333703, 0.3333333333333333703, 0.3333333333333333703, 0.3333333333333333703, 0.3333333333333333703, 0.3333333333333333703, 0.3333333333333333703, 0.3333333333333333703, 0.3333333333333333703, 0.3333333333333333703, 0.3333333333333333703, 0.3333333333333333703, 0.3333333333333333703, 0.3333333333333333703, 0.3333333333333333703, 0.3333333333333333703, 0.3333333333333333703, 0.3333333333333333703, 0.3333333333333333703),
 ( 0.3333333333333333703, 0.3333333333333333703, 0.3333333333333333703, 0.3333333333333333703, 0.3333333333333333703, 0.3333333333333333703, 0.3333333333333333703, 0.3333333333333333703, 0.3333333333333333703, 0.3333333333333333703, 0.3333333333333333703, 0.3333333333333333703, 0.3333333333333333703, 0.3333333333333333703, 0.3333333333333333703, 0.3333333333333333703, 0.3333333333333333703, 0.3333333333333333703, 0.3333333333333333703, 0.3333333333333333703, 0.3333333333333333703, 0.3333333333333333703, 0.3333333333333333703, 0.3333333333333333703, 0.3333333333333333703, 0.3333333333333333703, 0.3333333333333333703, 0.3333333333333333703, 0.3333333333333333703, 0.3333333333333333703, 0.3333333333333333703, 0.3333333333333333703, 0.3333333333333333703, 0.3333333333333333703, 0.3333333333333333703, 0.3333333333333333703, 0.3333333333333333703, 0.3333333333333333703),
 ( 1.000000000000000000, 1.000000000000000000, 1.000000000000000000, 1.000000000000000000, 1.000000000000000000, 1.000000000000000000, 1.000000000000000000, 1.000000000000000000, 1.000000000000000000, 1.000000000000000000, 1.000000000000000000, 1.000000000000000000, 1.000000000000000000, 1.000000000000000000, 1.000000000000000000, 1.000000000000000000, 1.000000000000000000, 1.000000000000000000, 1.000000000000000000, 1.000000000000000000, 1.000000000000000000, 1.000000000000000000, 1.000000000000000000, 1.000000000000000000, 1.000000000000000000, 1.000000000000000000, 1.000000000000000000, 1.000000000000000000, 1.000000000000000000, 1.000000000000000000, 1.000000000000000000, 1.000000000000000000, 1.000000000000000000, 1.000000000000000000, 1.000000000000000000, 1.000000000000000000, 1.000000000000000000, 1.000000000000000000) ) ) 
 REPRESENTATION_ITEM ( '' )  SURFACE ( )  );
#906=CARTESIAN_POINT ( 'NONE',  ( 8.599999999999996092, -50.00000000000000000, -1.639999999999997460 ) ) ;
#910=CARTESIAN_POINT ( 'NONE',  ( -11.03470001049236160, -47.20000000000001705, 2.958453039083849045 ) ) ;
#912=CARTESIAN_POINT ( 'NONE',  ( -9.116201041288242379, -50.00000000000000000, 7.005833569791151128 ) ) ;
#914=CARTESIAN_POINT ( 'NONE',  ( 8.324422814932072257, -47.20000000000001705, 2.231815450537910195 ) ) ;
#919=CARTESIAN_POINT ( 'NONE',  ( 8.530791689320604831, -50.00000000000000000, 1.124695299888175182 ) ) ;
#923=CARTESIAN_POINT ( 'NONE',  ( -9.959683570761574956, -50.00000000000000000, 5.743837162464267898 ) ) ;
#926=CARTESIAN_POINT ( 'NONE',  ( -11.29771452881884208, -50.53508261979052918, -1.297714528818841417 ) ) ;
#927=CARTESIAN_POINT ( 'NONE',  ( 4.331939449206418047, -52.79999999999999716, 7.514224851275111305 ) ) ;
#930=CARTESIAN_POINT ( 'NONE',  ( 8.596526774713712626, -50.00000000000000000, 0.2821220414049827596 ) ) ;
#939=CARTESIAN_POINT ( 'NONE',  ( 11.25335008359286704, -52.79999999999999716, 1.860476840074311911 ) ) ;
#940=CARTESIAN_POINT ( 'NONE',  ( 11.39999999999999680, -50.00000000000000000, -0.5466666666666269991 ) ) ;
#943=CARTESIAN_POINT ( 'NONE',  ( -6.877134118866001344, -52.79999999999999716, 5.285102517561345969 ) ) ;
#946=CARTESIAN_POINT ( 'NONE',  ( 8.599999999999996092, -50.00000000000000000, -0.5466666666666269991 ) ) ;
#948=CARTESIAN_POINT ( 'NONE',  ( 11.39999999999999680, -50.00000000000000000, -1.400000000003877254 ) ) ;
#956=CARTESIAN_POINT ( 'NONE',  ( 11.39999999999999680, -50.00000000000000000, -1.400000000003877254 ) ) ;
#958=CARTESIAN_POINT ( 'NONE',  ( -11.37702123033521850, -52.79999999999999716, 0.7471912688805021352 ) ) ;
#961=CARTESIAN_POINT ( 'NONE',  ( 2.982843918279706408, -52.79999999999999716, 11.10373667793903429 ) ) ;
#963=CARTESIAN_POINT ( 'NONE',  ( 8.599999999999996092, -50.00000000000000000, -1.639999999999997460 ) ) ;
#969=CARTESIAN_POINT ( 'NONE',  ( -11.39999999999999680, -47.20000000000001705, -1.093333333333363022 ) ) ;
#972=CARTESIAN_POINT ( 'NONE',  ( -11.39539595717873510, -52.79999999999999716, 0.3739757293043587949 ) ) ;
#973=CARTESIAN_POINT ( 'NONE',  ( 11.36325033731732503, -50.00000000000000000, 0.9334869871343942638 ) ) ;
#974=CARTESIAN_POINT ( 'NONE',  ( -9.597428871122712479, -51.34559595270263799, 0.3947853969006087649 ) ) ;
#975=CARTESIAN_POINT ( 'NONE',  ( -8.599999999999996092, -50.00000000000000000, -1.366666666666159768 ) ) ;
#977=CARTESIAN_POINT ( 'NONE',  ( 8.324422814932070480, -50.00000000000000000, 2.231815450537910639 ) ) ;
#984=CARTESIAN_POINT ( 'NONE',  ( 8.599999999999996092, -47.20000000000001705, -0.5466666666666269991 ) ) ;
#987=CARTESIAN_POINT ( 'NONE',  ( 11.20659079646779510, -50.71729705017420997, -1.206590796467808646 ) ) ;
#991=CARTESIAN_POINT ( 'NONE',  ( 11.03470001049091032, -52.79999999999999716, 2.958453039085699565 ) ) ;
#992=CARTESIAN_POINT ( 'NONE',  ( 11.39999532361432522, -50.00000000000000000, 0.1755699507458462760 ) ) ;
#994=CARTESIAN_POINT ( 'NONE',  ( -1.492255338562904265, -52.79999999999999716, 11.39999999999999680 ) ) ;
#996=ORIENTED_EDGE ( 'NONE', *, *, #1967, .T. ) ;
#1003=CARTESIAN_POINT ( 'NONE',  ( 11.64000000000000057, -50.00000000000000000, 1.399999999999999911 ) ) ;
#1008=CARTESIAN_POINT ( 'NONE',  ( 2.982843918279706408, -52.79999999999999716, 11.10373667793903429 ) ) ;
#1011=CARTESIAN_POINT ( 'NONE',  ( 4.331939449206418935, -50.00000000000000000, 7.514224851275112194 ) ) ;
#1019=CARTESIAN_POINT ( 'NONE',  ( -8.530791689320901483, -52.79999999999999716, 1.124695299888049504 ) ) ;
#1035=CARTESIAN_POINT ( 'NONE',  ( -7.513445500749800665, -50.00000000000000000, 4.333070140105378165 ) ) ;
#1039=CARTESIAN_POINT ( 'NONE',  ( 8.596526774713712626, -50.00000000000000000, 0.2821220414049827596 ) ) ;
#1045=CARTESIAN_POINT ( 'NONE',  ( 8.599999999999996092, -47.20000000000001705, -1.366666666666861873 ) ) ;
#1050=ADVANCED_FACE ( 'NONE', ( #2201 ), #9, .T. ) ;
#1052=CARTESIAN_POINT ( 'NONE',  ( 8.489369361306732031, -52.79999999999999716, 1.403517616196621409 ) ) ;
#1058=AXIS2_PLACEMENT_3D ( 'NONE', #3140, #2850, #1876 ) ;
#1064=CARTESIAN_POINT ( 'NONE',  ( 9.116201041286979390, -47.20000000000001705, 7.005833569791843907 ) ) ;
#1070=CARTESIAN_POINT ( 'NONE',  ( 2.250215587473118450, -50.00000000000000000, 8.376503107919017310 ) ) ;
#1078=CARTESIAN_POINT ( 'NONE',  ( 1.125736483477000061, -47.20000000000001705, 8.599999999999996092 ) ) ;
#1081=CARTESIAN_POINT ( 'NONE',  ( -8.452889752740315288, -50.00000000000000711, 1.586704117746376097 ) ) ;
#1086=CARTESIAN_POINT ( 'NONE',  ( 8.596526774713710850, -52.79999999999999716, 0.2821220414049827041 ) ) ;
#1092=CARTESIAN_POINT ( 'NONE',  ( 8.324422814932070480, -50.00000000000000000, 2.231815450537910639 ) ) ;
#1097=CARTESIAN_POINT ( 'NONE',  ( 9.116201041287551377, -50.00000000000000000, 7.005833569791843018 ) ) ;
#1099=CARTESIAN_POINT ( 'NONE',  ( -8.485280282859319456, -49.76857949351400379, 1.400000000000003020 ) ) ;
#1100=CARTESIAN_POINT ( 'NONE',  ( -1.125736483476999839, -50.00000000000000000, 8.599999999999996092 ) ) ;
#1103=CARTESIAN_POINT ( 'NONE',  ( 8.485280282859411827, -49.76857949351400379, 1.400000000000001243 ) ) ;
#1116=CARTESIAN_POINT ( 'NONE',  ( -11.39539595717873510, -52.79999999999999716, 0.3739757293043587949 ) ) ;
#1127=CARTESIAN_POINT ( 'NONE',  ( 9.959683570760009985, -47.20000000000001705, 5.743837162466679302 ) ) ;
#1131=CARTESIAN_POINT ( 'NONE',  ( -2.982843918280285944, -50.00000000000000000, 11.10373667793902541 ) ) ;
#1133=CYLINDRICAL_SURFACE ( 'NONE', #1058, 1.399999999999999911 ) ;
#1138=CARTESIAN_POINT ( 'NONE',  ( 9.595856219367004059, -48.65479562300421890, 0.3963015081148715257 ) ) ;
#1141=CARTESIAN_POINT ( 'NONE',  ( -7.005833569765055557, -50.00000000000000000, 9.116201041262108618 ) ) ;
#1145=CARTESIAN_POINT ( 'NONE',  ( -9.959683570761574956, -52.79999999999999716, 5.743837162464267898 ) ) ;
#1154=CARTESIAN_POINT ( 'NONE',  ( -8.600005876649037262, -50.00000000000000000, -0.2541998246238979520 ) ) ;
#1158=CARTESIAN_POINT ( 'NONE',  ( -10.81682914263834405, -47.20000000000001705, 3.675996170188739143 ) ) ;
#1163=CARTESIAN_POINT ( 'NONE',  ( -7.005833569765055557, -50.00000000000000000, 9.116201041262108618 ) ) ;
#1171=CARTESIAN_POINT ( 'NONE',  ( 8.599999999999996092, -50.00000000000000000, -1.639999999999997460 ) ) ;
#1176=CARTESIAN_POINT ( 'NONE',  ( 8.599999999999996092, -47.20000000000001705, -1.093333333333372126 ) ) ;
#1179=CARTESIAN_POINT ( 'NONE',  ( 9.959683570761143301, -52.79999999999999716, 5.743837162466679302 ) ) ;
#1181=CARTESIAN_POINT ( 'NONE',  ( 8.160064090060387798, -47.20000000000001705, 2.773119917860402239 ) ) ;
#1183=CARTESIAN_POINT ( 'NONE',  ( 11.33515354614431025, -49.56496474501408755, -1.335153546144312919 ) ) ;
#1191=CARTESIAN_POINT ( 'NONE',  ( 11.37702123033534995, -47.20000000000001705, 0.7471912688806705560 ) ) ;
#1194=CARTESIAN_POINT ( 'NONE',  ( 1.492255338562904265, -52.79999999999999716, 11.39999999999999680 ) ) ;
#1196=CARTESIAN_POINT ( 'NONE',  ( 8.160064090060387798, -50.00000000000000000, 2.773119917860402239 ) ) ;
#1205=CARTESIAN_POINT ( 'NONE',  ( 11.38628138490143016, -50.22360298513552124, -1.386281384901437264 ) ) ;
#1207=CARTESIAN_POINT ( 'NONE',  ( 7.005833569765714586, -50.00000000000000000, 9.116201041261451365 ) ) ;
#1210=CARTESIAN_POINT ( 'NONE',  ( 8.599999999999996092, -52.79999999999999716, -0.5466666666666269991 ) ) ;
#1213=CARTESIAN_POINT ( 'NONE',  ( 4.331939449206418935, -50.00000000000000000, 7.514224851275112194 ) ) ;
#1219=CARTESIAN_POINT ( 'NONE',  ( -6.877134118866000456, -50.00000000000000000, 5.285102517561346858 ) ) ;
#1224=CARTESIAN_POINT ( 'NONE',  ( -11.03470001049179494, -52.79999999999999716, 2.958453039083849045 ) ) ;
#1225=CARTESIAN_POINT ( 'NONE',  ( 7.005833569765714586, -50.00000000000000000, 9.116201041261451365 ) ) ;
#1226=CARTESIAN_POINT ( 'NONE',  ( -11.03475136337292639, -50.94770623811574239, -1.034751363372938160 ) ) ;
#1227=CARTESIAN_POINT ( 'NONE',  ( 11.39999999999999680, -52.79999999999999716, -1.639999999999997460 ) ) ;
#1228=ORIENTED_EDGE ( 'NONE', *, *, #1967, .F. ) ;
#1229=CARTESIAN_POINT ( 'NONE',  ( 7.513445500750180805, -50.00000000000000000, 4.333070140107198043 ) ) ;
#1233=CARTESIAN_POINT ( 'NONE',  ( -11.39999999999999680, -47.20000000000001705, -1.639999999999997460 ) ) ;
#1234=CARTESIAN_POINT ( 'NONE',  ( -11.40000000000000036, -49.88862030549578463, -1.400000000000000355 ) ) ;
#1237=CARTESIAN_POINT ( 'NONE',  ( 9.920087608940491464, -51.40000000000001279, 0.07988930269788889482 ) ) ;
#1238=CARTESIAN_POINT ( 'NONE',  ( 9.116201041288118034, -52.79999999999999716, 7.005833569791843907 ) ) ;
#1239=CARTESIAN_POINT ( 'NONE',  ( 5.742338339643763945, -50.00000000000000000, 9.960716663318306630 ) ) ;
#1241=CARTESIAN_POINT ( 'NONE',  ( -8.599999999999996092, -52.79999999999999716, -1.639999999999997460 ) ) ;
#1243=CARTESIAN_POINT ( 'NONE',  ( -6.877134118866001344, -47.20000000000001705, 5.285102517561345969 ) ) ;
#1244=PRODUCT_CONTEXT ( 'NONE', #3220, 'mechanical' ) ;
#1253=CARTESIAN_POINT ( 'NONE',  ( 11.39999532361432522, -52.79999999999999716, 0.1755699507458462760 ) ) ;
#1254=CARTESIAN_POINT ( 'NONE',  ( 11.37702123033542279, -50.00000000000000000, 0.7471912688806704450 ) ) ;
#1255=( LENGTH_UNIT ( ) NAMED_UNIT ( * ) SI_UNIT ( .MILLI., .METRE. ) );
#1256=CARTESIAN_POINT ( 'NONE',  ( -8.582665138674013150, -50.00000000000000000, 0.5636706063486749407 ) ) ;
#1263=CARTESIAN_POINT ( 'NONE',  ( -9.999999999999998224, -48.60000000000000142, 1.734719587726169024E-19 ) ) ;
#1268=CARTESIAN_POINT ( 'NONE',  ( 8.489369361306732031, -50.00000000000000000, 1.403517616196621409 ) ) ;
#1270=( NAMED_UNIT ( * ) PLANE_ANGLE_UNIT ( ) SI_UNIT ( $, .RADIAN. ) );
#1275=ORIENTED_EDGE ( 'NONE', *, *, #2410, .T. ) ;
#1282=CARTESIAN_POINT ( 'NONE',  ( 8.502540660504635639, -50.22987518539597573, 1.385387373903631314 ) ) ;
#1283=CARTESIAN_POINT ( 'NONE',  ( 8.582665138674004268, -50.00000000000000000, 0.5636706063485154017 ) ) ;
#1290=VERTEX_POINT ( 'NONE', #1611 ) ;
#1292=CARTESIAN_POINT ( 'NONE',  ( 7.513445500750181694, -47.20000000000001705, 4.333070140107198043 ) ) ;
#1293=EDGE_LOOP ( 'NONE', ( #1388, #2887, #514, #3110, #2636, #1559 ) ) ;
#1301=CARTESIAN_POINT ( 'NONE',  ( -8.582665138674013150, -50.00000000000000000, 0.5636706063486749407 ) ) ;
#1307=CARTESIAN_POINT ( 'NONE',  ( -8.530791689320901483, -50.00000000000000000, 1.124695299888049504 ) ) ;
#1313=CARTESIAN_POINT ( 'NONE',  ( -11.40000778997679198, -47.20000000000001705, -0.2924664341913127408 ) ) ;
#1318=CARTESIAN_POINT ( 'NONE',  ( -8.572276570256935457, -52.79999999999999716, 0.7042094815226510596 ) ) ;
#1323=CARTESIAN_POINT ( 'NONE',  ( 8.489369361306732031, -50.00000000000000000, 1.403517616196621409 ) ) ;
#1324=CARTESIAN_POINT ( 'NONE',  ( 5.285102517541700351, -50.00000000000000000, 6.877134118846478295 ) ) ;
#1328=CARTESIAN_POINT ( 'NONE',  ( -9.959683570761574956, -47.20000000000001705, 5.743837162464267898 ) ) ;
#1332=CARTESIAN_POINT ( 'NONE',  ( -8.324422814933019055, -50.00000000000000000, 2.231815450536601464 ) ) ;
#1335=CARTESIAN_POINT ( 'NONE',  ( -8.599996472200352571, -50.00000000000000000, 0.1525981975067654262 ) ) ;
#1340=CARTESIAN_POINT ( 'NONE',  ( 8.452889752740453844, -50.00000000000000000, 1.586704117746243314 ) ) ;
#1343=CARTESIAN_POINT ( 'NONE',  ( 8.599999999999996092, -47.20000000000001705, -1.093333333333372126 ) ) ;
#1348=CARTESIAN_POINT ( 'NONE',  ( -4.331939449206426929, -50.00000000000000000, 7.514224851276241957 ) ) ;
#1352=CARTESIAN_POINT ( 'NONE',  ( 9.920079092145082100, -48.60000000000001563, 0.07989781697635986446 ) ) ;
#1362=CARTESIAN_POINT ( 'NONE',  ( -11.39999532361432522, -52.79999999999999716, 0.1755699507458657049 ) ) ;
#1366=CARTESIAN_POINT ( 'NONE',  ( 2.250215587473118450, -50.00000000000000000, 8.376503107919017310 ) ) ;
#1367=ORIENTED_EDGE ( 'NONE', *, *, #697, .T. ) ;
#1370=CARTESIAN_POINT ( 'NONE',  ( 8.599999999999996092, -50.00000000000000000, -1.093333333333372126 ) ) ;
#1371=EDGE_LOOP ( 'NONE', ( #885, #2968, #1275, #1228, #2310, #139 ) ) ;
#1377=CARTESIAN_POINT ( 'NONE',  ( -2.982843918280285944, -47.20000000000001705, 11.10373667793902541 ) ) ;
#1379=( GEOMETRIC_REPRESENTATION_CONTEXT ( 3 ) GLOBAL_UNCERTAINTY_ASSIGNED_CONTEXT ( ( #1501 ) ) GLOBAL_UNIT_ASSIGNED_CONTEXT ( ( #2622, #2894, #880 ) ) REPRESENTATION_CONTEXT ( 'NONE', 'WORKASPACE' ) );
#1381=CARTESIAN_POINT ( 'NONE',  ( -11.30825875095987421, -52.79999999999999716, 1.490875164968288757 ) ) ;
#1388=ORIENTED_EDGE ( 'NONE', *, *, #507, .F. ) ;
#1390=( NAMED_UNIT ( * ) SI_UNIT ( $, .STERADIAN. ) SOLID_ANGLE_UNIT ( ) );
#1392=CARTESIAN_POINT ( 'NONE',  ( -11.39999999999999680, -50.00000000000000000, -0.5466666666666361030 ) ) ;
#1393=CARTESIAN_POINT ( 'NONE',  ( -11.39999999999999680, -50.00000000000000000, -1.013333333333681141 ) ) ;
#1395=CARTESIAN_POINT ( 'NONE',  ( -11.03470001049179494, -52.79999999999999716, 2.958453039083849045 ) ) ;
#1401=ADVANCED_BREP_SHAPE_REPRESENTATION ( '', ( #1612, #1692 ), #1379 ) ;
#1404=ORIENTED_EDGE ( 'NONE', *, *, #1442, .T. ) ;
#1406=SURFACE_SIDE_STYLE ('',( #1886 ) ) ;
#1407=CARTESIAN_POINT ( 'NONE',  ( -11.36325033731739076, -47.20000000000001705, 0.9334869871344717573 ) ) ;
#1408=CARTESIAN_POINT ( 'NONE',  ( -7.005833569765055557, -50.00000000000000000, 9.116201041262108618 ) ) ;
#1412=CARTESIAN_POINT ( 'NONE',  ( 11.03470001049119453, -50.00000000000000000, 2.958453039085983338 ) ) ;
#1418=ORIENTED_EDGE ( 'NONE', *, *, #2173, .F. ) ;
#1419=CARTESIAN_POINT ( 'NONE',  ( 8.599999999999996092, -50.00000000000000000, -1.093333333333372126 ) ) ;
#1423=CARTESIAN_POINT ( 'NONE',  ( 7.005833569766282132, -47.20000000000001705, 9.116201041261453142 ) ) ;
#1426=CARTESIAN_POINT ( 'NONE',  ( -9.920087608911693167, -51.39999999999999858, 0.07988930266963500948 ) ) ;
#1428=CARTESIAN_POINT ( 'NONE',  ( 11.39999999999999680, -50.00000000000000000, -1.366666666666861873 ) ) ;
#1429=ORIENTED_EDGE ( 'NONE', *, *, #1474, .F. ) ;
#1430=CARTESIAN_POINT ( 'NONE',  ( -8.324422814933019055, -47.20000000000001705, 2.231815450536601020 ) ) ;
#1435=CARTESIAN_POINT ( 'NONE',  ( 1.125736483476999839, -50.00000000000000000, 8.599999999999996092 ) ) ;
#1436=CARTESIAN_POINT ( 'NONE',  ( -11.33515354614430670, -49.56496474501410887, -1.335153546144310699 ) ) ;
#1437=CARTESIAN_POINT ( 'NONE',  ( 10.31604092329498989, -51.37342103705936580, -0.3160374682705313631 ) ) ;
#1440=CARTESIAN_POINT ( 'NONE',  ( 2.982843918280841500, -47.20000000000001705, 11.10373667793903074 ) ) ;
#1442=EDGE_CURVE ( 'NONE', #2378, #890, #2873, .T. ) ;
#1443=CARTESIAN_POINT ( 'NONE',  ( -10.62090117298859759, -51.26516722440712925, -0.6209000891238662945 ) ) ;
#1444=CARTESIAN_POINT ( 'NONE',  ( 11.39999999999999680, -52.79999999999999716, -1.093333333333372126 ) ) ;
#1446=CARTESIAN_POINT ( 'NONE',  ( -8.489369361306263073, -50.00000000000000000, 1.403517616197273554 ) ) ;
#1450=CARTESIAN_POINT ( 'NONE',  ( 6.877134118866902845, -50.00000000000000000, 5.285102517562147995 ) ) ;
#1454=CARTESIAN_POINT ( 'NONE',  ( 2.982843918280273510, -50.00000000000000000, 11.10373667793903252 ) ) ;
#1455=CARTESIAN_POINT ( 'NONE',  ( 11.39999999999999680, -50.00000000000000000, -1.206666666669127919 ) ) ;
#1458=CARTESIAN_POINT ( 'NONE',  ( 8.582665138674004268, -52.79999999999999716, 0.5636706063485154017 ) ) ;
#1460=CARTESIAN_POINT ( 'NONE',  ( -8.599996472200352571, -47.20000000000001705, 0.1525981975067654817 ) ) ;
#1468=CARTESIAN_POINT ( 'NONE',  ( -4.331939449206426929, -50.00000000000000000, 7.514224851276241957 ) ) ;
#1472=CARTESIAN_POINT ( 'NONE',  ( -11.39999999999999680, -52.79999999999999716, -1.093333333333363022 ) ) ;
#1474=EDGE_CURVE ( 'NONE', #2378, #661, #2444, .T. ) ;
#1476=CARTESIAN_POINT ( 'NONE',  ( 11.37702123033549384, -52.79999999999999716, 0.7471912688806703340 ) ) ;
#1480=CARTESIAN_POINT ( 'NONE',  ( -4.331939449206426929, -50.00000000000000000, 7.514224851276241957 ) ) ;
#1482=CARTESIAN_POINT ( 'NONE',  ( 11.29810924534245231, -49.46572717680115261, -1.298109245342459639 ) ) ;
#1486=CARTESIAN_POINT ( 'NONE',  ( 8.582665138674004268, -47.20000000000001705, 0.5636706063485154017 ) ) ;
#1490=CARTESIAN_POINT ( 'NONE',  ( 10.76674801461901687, -51.18483196047734651, -0.7667480146190301937 ) ) ;
#1491=CARTESIAN_POINT ( 'NONE',  ( 8.768448914935811800, -50.81504429929027822, 1.156277961913187990 ) ) ;
#1492=CARTESIAN_POINT ( 'NONE',  ( 5.742338339643763945, -50.00000000000000000, 9.960716663318306630 ) ) ;
#1493=CARTESIAN_POINT ( 'NONE',  ( 9.959683570760574867, -50.00000000000000000, 5.743837162466680191 ) ) ;
#1496=CARTESIAN_POINT ( 'NONE',  ( 7.005833569765147040, -52.79999999999999716, 9.116201041261453142 ) ) ;
#1498=CARTESIAN_POINT ( 'NONE',  ( 7.513445500750181694, -47.20000000000001705, 4.333070140107198043 ) ) ;
#1501=UNCERTAINTY_MEASURE_WITH_UNIT (LENGTH_MEASURE( 1.000000000000000082E-05 ), #2622, 'distance_accuracy_value', 'NONE');
#1505=CARTESIAN_POINT ( 'NONE',  ( 11.39999999999999680, -50.00000000000000000, -1.366666666666861873 ) ) ;
#1507=CARTESIAN_POINT ( 'NONE',  ( -8.596526774713707297, -50.00000000000000000, 0.2821220414048196679 ) ) ;
#1521=CARTESIAN_POINT ( 'NONE',  ( -8.600005876649037262, -52.79999999999999716, -0.2541998246238979520 ) ) ;
#1540=CARTESIAN_POINT ( 'NONE',  ( 8.324422814932072257, -52.79999999999999716, 2.231815450537910195 ) ) ;
#1544=CARTESIAN_POINT ( 'NONE',  ( 6.877134118866902845, -50.00000000000000000, 5.285102517562147995 ) ) ;
#1548=SHAPE_DEFINITION_REPRESENTATION ( #3134, #2799 ) ;
#1549=CARTESIAN_POINT ( 'NONE',  ( 2.250215587473118450, -47.20000000000001705, 8.376503107919017310 ) ) ;
#1554=CARTESIAN_POINT ( 'NONE',  ( 9.597428871123410588, -51.34559595270280852, 0.3947853968998988328 ) ) ;
#1555=CARTESIAN_POINT ( 'NONE',  ( -2.250215587473127332, -50.00000000000000000, 8.376503107917878665 ) ) ;
#1559=ORIENTED_EDGE ( 'NONE', *, *, #15, .T. ) ;
#1561=CARTESIAN_POINT ( 'NONE',  ( 1.492255338562904265, -47.20000000000001705, 11.39999999999999680 ) ) ;
#1568=CARTESIAN_POINT ( 'NONE',  ( -8.160064090060583197, -50.00000000000000000, 2.773119917861301964 ) ) ;
#1570=B_SPLINE_CURVE_WITH_KNOTS ( 'NONE', 3,
 ( #379, #1103, #2939, #2433, #1665, #2908, #159, #1138, #345, #681, #1352, #1683 ),
 .UNSPECIFIED., .F., .F.,
 ( 4, 2, 2, 2, 2, 4 ),
 ( 0.002704438958034565722, 0.003382491784585806537, 0.004060544611137047351, 0.004738597437688288165, 0.005077623850963906837, 0.005416650264239525510 ),
 .UNSPECIFIED. ) ;
#1574=CARTESIAN_POINT ( 'NONE',  ( 2.250215587473118450, -50.00000000000000000, 8.376503107919017310 ) ) ;
#1578=CARTESIAN_POINT ( 'NONE',  ( 11.03470001049147697, -47.20000000000001705, 2.958453039086267111 ) ) ;
#1585=CARTESIAN_POINT ( 'NONE',  ( 5.285102517541700351, -50.00000000000000000, 6.877134118846478295 ) ) ;
#1596=CARTESIAN_POINT ( 'NONE',  ( -8.599999999999996092, -47.20000000000001705, -1.366666666666159546 ) ) ;
#1599=CARTESIAN_POINT ( 'NONE',  ( -6.877134118866000456, -50.00000000000000000, 5.285102517561346858 ) ) ;
#1603=CARTESIAN_POINT ( 'NONE',  ( -6.877134118866001344, -52.79999999999999716, 5.285102517561345969 ) ) ;
#1609=CARTESIAN_POINT ( 'NONE',  ( -11.36325033731746004, -50.00000000000000000, 0.9334869871344717573 ) ) ;
#1611=CARTESIAN_POINT ( 'NONE',  ( 9.999999999999976907, -48.60000000000000142, -1.084199742356775455E-20 ) ) ;
#1612=MANIFOLD_SOLID_BREP ( 'Sweep1', #141 ) ;
#1613=CARTESIAN_POINT ( 'NONE',  ( -11.36325033731746004, -50.00000000000000000, 0.9334869871344717573 ) ) ;
#1615=CARTESIAN_POINT ( 'NONE',  ( -9.999999999999998224, -48.60000000000000142, 1.734719587726169024E-19 ) ) ;
#1619=CARTESIAN_POINT ( 'NONE',  ( 11.64000000000000057, -50.00000000000000000, -1.399999999999999911 ) ) ;
#1622=STYLED_ITEM('',(#3293),#1612);
#1625=CARTESIAN_POINT ( 'NONE',  ( -11.37702123033536061, -47.20000000000001705, 0.7471912688805021352 ) ) ;
#1629=CARTESIAN_POINT ( 'NONE',  ( 11.39539595717853082, -50.00000000000000000, 0.3739757293042009212 ) ) ;
#1640=CARTESIAN_POINT ( 'NONE',  ( -5.742338339643776379, -47.20000000000001705, 9.960716663318299524 ) ) ;
#1644=CARTESIAN_POINT ( 'NONE',  ( 11.39999532361432522, -50.00000000000000000, 0.1755699507458462760 ) ) ;
#1651=CARTESIAN_POINT ( 'NONE',  ( 8.489369361306732031, -50.00000000000000000, 1.403517616196621409 ) ) ;
#1654=FACE_OUTER_BOUND ( 'NONE', #1371, .T. ) ;
#1655=CARTESIAN_POINT ( 'NONE',  ( 11.30825875096014066, -47.20000000000001705, 1.490875164968454625 ) ) ;
#1656=CARTESIAN_POINT ( 'NONE',  ( -10.81682914263834405, -50.00000000000000000, 3.675996170188739143 ) ) ;
#1658=CARTESIAN_POINT ( 'NONE',  ( 11.39999999999999680, -50.00000000000000000, -1.639999999999997460 ) ) ;
#1660=CARTESIAN_POINT ( 'NONE',  ( -8.904708611508519667, -49.04279439154561970, 1.036389030864862448 ) ) ;
#1664=CARTESIAN_POINT ( 'NONE',  ( 8.600005876649037262, -50.00000000000000000, -0.2541998246239300374 ) ) ;
#1665=CARTESIAN_POINT ( 'NONE',  ( 8.904708611508466376, -49.04279439154559128, 1.036389030864799832 ) ) ;
#1668=CARTESIAN_POINT ( 'NONE',  ( -7.005833569763921354, -47.20000000000001705, 9.116201041262108618 ) ) ;
#1670=CARTESIAN_POINT ( 'NONE',  ( -8.485280282859317680, -50.00000000000000000, 1.400000000000003020 ) ) ;
#1672=CARTESIAN_POINT ( 'NONE',  ( -11.39999999999999680, -50.00000000000000000, -1.366666666666159768 ) ) ;
#1675=CARTESIAN_POINT ( 'NONE',  ( 8.582665138674004268, -47.20000000000001705, 0.5636706063485154017 ) ) ;
#1682=CARTESIAN_POINT ( 'NONE',  ( -8.599999999999996092, -47.20000000000001705, -1.639999999999997460 ) ) ;
#1683=CARTESIAN_POINT ( 'NONE',  ( 9.999999999999976907, -48.60000000000000142, -1.084199742356775455E-20 ) ) ;
#1684=CARTESIAN_POINT ( 'NONE',  ( 10.97094949647942030, -51.01251636945240620, -0.9709494964794326277 ) ) ;
#1686=CARTESIAN_POINT ( 'NONE',  ( -11.40000778997679198, -47.20000000000001705, -0.2924664341913127408 ) ) ;
#1691=CARTESIAN_POINT ( 'NONE',  ( 2.250215587473118450, -52.79999999999999716, 8.376503107919017310 ) ) ;
#1692=AXIS2_PLACEMENT_3D ( 'NONE', #3075, #2051, #2104 ) ;
#1694=CARTESIAN_POINT ( 'NONE',  ( 8.572276570257084671, -50.00000000000000000, 0.7042094815225934390 ) ) ;
#1695=CARTESIAN_POINT ( 'NONE',  ( 11.03726195774814833, -49.04331167652343026, -1.037261957748134344 ) ) ;
#1696=VERTEX_POINT ( 'NONE', #381 ) ;
#1702=CARTESIAN_POINT ( 'NONE',  ( 11.37702123033542279, -50.00000000000000000, 0.7471912688806704450 ) ) ;
#1704=CARTESIAN_POINT ( 'NONE',  ( -8.485280282859321233, -50.11569792258599421, 1.400000000000003242 ) ) ;
#1705=CARTESIAN_POINT ( 'NONE',  ( 8.572276570257082895, -52.79999999999999716, 0.7042094815225934390 ) ) ;
#1707=CARTESIAN_POINT ( 'NONE',  ( 8.489369361306732031, -50.00000000000000000, 1.403517616196621409 ) ) ;
#1713=CARTESIAN_POINT ( 'NONE',  ( -8.582665138674013150, -50.00000000000000000, 0.5636706063486749407 ) ) ;
#1714=LINE ( 'NONE', #1003, #898 ) ;
#1719=CARTESIAN_POINT ( 'NONE',  ( 9.959683570760574867, -50.00000000000000000, 5.743837162466680191 ) ) ;
#1720=CARTESIAN_POINT ( 'NONE',  ( 10.81682914263883610, -50.00000000000000000, 3.675996170187548540 ) ) ;
#1722=CARTESIAN_POINT ( 'NONE',  ( 8.599999999999996092, -52.79999999999999716, -1.366666666666861873 ) ) ;
#1724=CARTESIAN_POINT ( 'NONE',  ( -5.285102517542626721, -47.20000000000001705, 6.877134118847253674 ) ) ;
#1730=CARTESIAN_POINT ( 'NONE',  ( 6.877134118866901957, -47.20000000000001705, 5.285102517562147995 ) ) ;
#1734=CARTESIAN_POINT ( 'NONE',  ( -8.599999999999996092, -50.00000000000000000, -1.639999999999997460 ) ) ;
#1735=CARTESIAN_POINT ( 'NONE',  ( 11.30825875096042310, -52.79999999999999716, 1.490875164968454625 ) ) ;
#1736=CARTESIAN_POINT ( 'NONE',  ( 11.40000778997679021, -50.00000000000000000, -0.2924664341912772692 ) ) ;
#1737=CARTESIAN_POINT ( 'NONE',  ( -11.33527052789730405, -50.43454227690136094, -1.335270527897301385 ) ) ;
#1738=B_SPLINE_CURVE_WITH_KNOTS ( 'NONE', 3,
 ( #369, #3135, #1393, #2143, #869, #164, #3150, #3197, #1609, #2655, #3167, #2914, #1656, #2669, #399, #1408, #2944, #436, #2007, #3262, #1976, #1239, #1225, #2979, #1493, #1720, #750, #484, #2994, #973, #1254, #686, #992, #1736, #940, #451, #1455, #2489 ),
 .UNSPECIFIED., .F., .F.,
 ( 4, 2, 2, 2, 2, 2, 2, 2, 2, 2, 2, 2, 2, 2, 2, 2, 2, 2, 4 ),
 ( -0.04443856763921243819, -0.02602830390294905150, 0.000000000000000000, 0.01562500000000000694, 0.03125000000000000694, 0.06250000000000000000, 0.1250000000000000000, 0.2500000000000000000, 0.3750000000000000000, 0.4999999999999999445, 0.6250000000000000000, 0.7500000000000000000, 0.8750000000000000000, 0.9374999999999998890, 0.9687500000000001110, 0.9843750000000001110, 1.000000000000000000, 1.026028303902949190, 1.044438567639293325 ),
 .UNSPECIFIED. ) ;
#1741=CARTESIAN_POINT ( 'NONE',  ( -8.160064090060583197, -52.79999999999999716, 2.773119917861301520 ) ) ;
#1744=CARTESIAN_POINT ( 'NONE',  ( 1.125736483476999839, -50.00000000000000000, 8.599999999999996092 ) ) ;
#1747=CARTESIAN_POINT ( 'NONE',  ( -10.61784491273703246, -48.73341048396267894, -0.6178437967800078923 ) ) ;
#1750=CARTESIAN_POINT ( 'NONE',  ( -8.599999999999996092, -52.79999999999999716, -1.639999999999997460 ) ) ;
#1753=CARTESIAN_POINT ( 'NONE',  ( -2.250215587473127332, -52.79999999999999716, 8.376503107917878665 ) ) ;
#1765=CARTESIAN_POINT ( 'NONE',  ( -8.599999999999996092, -52.79999999999999716, -1.366666666666159546 ) ) ;
#1768=CARTESIAN_POINT ( 'NONE',  ( -4.331939449206426929, -50.00000000000000000, 7.514224851276241957 ) ) ;
#1780=CARTESIAN_POINT ( 'NONE',  ( 4.331939449206418047, -52.79999999999999716, 7.514224851275111305 ) ) ;
#1784=CARTESIAN_POINT ( 'NONE',  ( -5.285102517542626721, -50.00000000000000000, 6.877134118847252786 ) ) ;
#1788=CARTESIAN_POINT ( 'NONE',  ( -8.489369361306263073, -47.20000000000001705, 1.403517616197273554 ) ) ;
#1798=CARTESIAN_POINT ( 'NONE',  ( -8.572276570256935457, -50.00000000000000000, 0.7042094815226510596 ) ) ;
#1801=CARTESIAN_POINT ( 'NONE',  ( 8.572276570257084671, -50.00000000000000000, 0.7042094815225934390 ) ) ;
#1806=CARTESIAN_POINT ( 'NONE',  ( -11.39539595717859299, -47.20000000000001705, 0.3739757293043587949 ) ) ;
#1813=CARTESIAN_POINT ( 'NONE',  ( -1.125736483477000061, -52.79999999999999716, 8.599999999999996092 ) ) ;
#1817=CARTESIAN_POINT ( 'NONE',  ( -2.250215587473127332, -50.00000000000000000, 8.376503107917878665 ) ) ;
#1818=CARTESIAN_POINT ( 'NONE',  ( 8.469856736028367195, -50.00000000000000000, 1.493482969799619031 ) ) ;
#1822=CARTESIAN_POINT ( 'NONE',  ( -8.160064090060583197, -47.20000000000001705, 2.773119917861301520 ) ) ;
#1830=CARTESIAN_POINT ( 'NONE',  ( -1.125736483476999839, -50.00000000000000000, 8.599999999999996092 ) ) ;
#1835=DIRECTION ( 'NONE',  ( 0.000000000000000000, 0.000000000000000000, 1.000000000000000000 ) ) ;
#1836=EDGE_LOOP ( 'NONE', ( #203, #2891, #556, #860, #1418, #996 ) ) ;
#1838=CARTESIAN_POINT ( 'NONE',  ( -8.324422814933019055, -47.20000000000001705, 2.231815450536601020 ) ) ;
#1845=CARTESIAN_POINT ( 'NONE',  ( -7.513445500749801553, -52.79999999999999716, 4.333070140105379942 ) ) ;
#1855=CARTESIAN_POINT ( 'NONE',  ( 2.982843918280273510, -50.00000000000000000, 11.10373667793903252 ) ) ;
#1867=PRESENTATION_STYLE_ASSIGNMENT (( #2406 ) ) ;
#1869=CARTESIAN_POINT ( 'NONE',  ( -11.39999999999999680, -50.00000000000000000, -1.366666666666159768 ) ) ;
#1873=CARTESIAN_POINT ( 'NONE',  ( 11.40000778997679021, -50.00000000000000000, -0.2924664341912772692 ) ) ;
#1876=DIRECTION ( 'NONE',  ( 0.000000000000000000, 0.000000000000000000, 1.000000000000000000 ) ) ;
#1886=SURFACE_STYLE_FILL_AREA ( #2157 ) ;
#1887=CARTESIAN_POINT ( 'NONE',  ( -5.742338339643776379, -50.00000000000000000, 9.960716663318299524 ) ) ;
#1892=CARTESIAN_POINT ( 'NONE',  ( -11.30825875096001454, -50.00000000000000000, 1.490875164968288757 ) ) ;
#1899=CARTESIAN_POINT ( 'NONE',  ( 2.250215587473118450, -50.00000000000000000, 8.376503107919017310 ) ) ;
#1904=( NAMED_UNIT ( * ) PLANE_ANGLE_UNIT ( ) SI_UNIT ( $, .RADIAN. ) );
#1906=CARTESIAN_POINT ( 'NONE',  ( -1.492255338562904043, -50.00000000000000000, 11.39999999999999680 ) ) ;
#1910=CARTESIAN_POINT ( 'NONE',  ( 11.40000778997679198, -47.20000000000001705, -0.2924664341912773247 ) ) ;
#1916=CARTESIAN_POINT ( 'NONE',  ( 8.572276570257084671, -50.00000000000000000, 0.7042094815225934390 ) ) ;
#1917=CARTESIAN_POINT ( 'NONE',  ( 8.600005876649037262, -50.00000000000000000, -0.2541998246239300374 ) ) ;
#1921=CARTESIAN_POINT ( 'NONE',  ( -11.37702123033528778, -50.00000000000000000, 0.7471912688805022462 ) ) ;
#1925=CARTESIAN_POINT ( 'NONE',  ( -5.742338339643776379, -50.00000000000000000, 9.960716663318299524 ) ) ;
#1927=CARTESIAN_POINT ( 'NONE',  ( 8.489369361306732031, -47.20000000000001705, 1.403517616196621409 ) ) ;
#1937=CARTESIAN_POINT ( 'NONE',  ( 8.599999999999996092, -47.20000000000001705, -0.5466666666666269991 ) ) ;
#1940=CARTESIAN_POINT ( 'NONE',  ( -11.39999999999999680, -50.00000000000000000, -1.400000000000000133 ) ) ;
#1941=CARTESIAN_POINT ( 'NONE',  ( 6.877134118866901957, -52.79999999999999716, 5.285102517562147995 ) ) ;
#1944=CARTESIAN_POINT ( 'NONE',  ( -6.877134118866000456, -50.00000000000000000, 5.285102517561346858 ) ) ;
#1947=CARTESIAN_POINT ( 'NONE',  ( 10.61784491273702180, -48.73341048396265052, -0.6178437967800165520 ) ) ;
#1948=ADVANCED_FACE ( 'NONE', ( #1654 ), #901, .T. ) ;
#1956=CARTESIAN_POINT ( 'NONE',  ( 7.005833569765147040, -52.79999999999999716, 9.116201041261453142 ) ) ;
#1959=CARTESIAN_POINT ( 'NONE',  ( -9.199433601068362165, -51.18229052107376020, 0.7695943483570758525 ) ) ;
#1961=CARTESIAN_POINT ( 'NONE',  ( 5.285102517541700351, -52.79999999999999716, 6.877134118846478295 ) ) ;
#1964=CARTESIAN_POINT ( 'NONE',  ( -8.599999999999996092, -47.20000000000001705, -1.366666666666159546 ) ) ;
#1967=EDGE_CURVE ( 'NONE', #403, #1290, #1570, .T. ) ;
#1975=CARTESIAN_POINT ( 'NONE',  ( 11.03470001049119453, -50.00000000000000000, 2.958453039085983338 ) ) ;
#1976=CARTESIAN_POINT ( 'NONE',  ( 2.982843918280273510, -50.00000000000000000, 11.10373667793903252 ) ) ;
#1978=CARTESIAN_POINT ( 'NONE',  ( -5.285102517542626721, -52.79999999999999716, 6.877134118847253674 ) ) ;
#1980=CARTESIAN_POINT ( 'NONE',  ( 8.530791689320604831, -50.00000000000000000, 1.124695299888175182 ) ) ;
#1985=CARTESIAN_POINT ( 'NONE',  ( -11.36325033731739076, -47.20000000000001705, 0.9334869871344717573 ) ) ;
#1989=CARTESIAN_POINT ( 'NONE',  ( -8.600005876649037262, -50.00000000000000000, -0.2541998246238979520 ) ) ;
#1990=CARTESIAN_POINT ( 'NONE',  ( 11.40000778997679021, -50.00000000000000000, -0.2924664341912772692 ) ) ;
#1992=CARTESIAN_POINT ( 'NONE',  ( -8.609154349732479616, -50.54332563323215055, 1.294262817215226846 ) ) ;
#1993=CARTESIAN_POINT ( 'NONE',  ( 11.39999532361432522, -52.79999999999999716, 0.1755699507458462760 ) ) ;
#1995=CARTESIAN_POINT ( 'NONE',  ( 5.285102517541700351, -47.20000000000001705, 6.877134118846478295 ) ) ;
#2001=CARTESIAN_POINT ( 'NONE',  ( 8.572276570257082895, -47.20000000000001705, 0.7042094815225934390 ) ) ;
#2002=CARTESIAN_POINT ( 'NONE',  ( -11.03726195774814478, -49.04331167652343026, -1.037261957748144114 ) ) ;
#2006=CARTESIAN_POINT ( 'NONE',  ( 9.959683570761143301, -52.79999999999999716, 5.743837162466679302 ) ) ;
#2007=CARTESIAN_POINT ( 'NONE',  ( -1.492255338562904043, -50.00000000000000000, 11.39999999999999680 ) ) ;
#2011=CARTESIAN_POINT ( 'NONE',  ( -8.599999999999996092, -52.79999999999999716, -0.5466666666666361030 ) ) ;
#2023=CARTESIAN_POINT ( 'NONE',  ( 11.39999999999999680, -52.79999999999999716, -1.093333333333372126 ) ) ;
#2026=CARTESIAN_POINT ( 'NONE',  ( 5.285102517541700351, -50.00000000000000000, 6.877134118846478295 ) ) ;
#2032=UNCERTAINTY_MEASURE_WITH_UNIT (LENGTH_MEASURE( 1.000000000000000082E-05 ), #382, 'distance_accuracy_value', 'NONE');
#2036=CARTESIAN_POINT ( 'NONE',  ( -8.599999999999996092, -50.00000000000000000, -1.639999999999997460 ) ) ;
#2048=CARTESIAN_POINT ( 'NONE',  ( 8.485280282859413603, -50.00000000000000000, 1.400000000000001021 ) ) ;
#2049=CARTESIAN_POINT ( 'NONE',  ( 8.599999999999996092, -52.79999999999999716, -1.639999999999997460 ) ) ;
#2051=DIRECTION ( 'NONE',  ( 0.000000000000000000, 0.000000000000000000, 1.000000000000000000 ) ) ;
#2052=CARTESIAN_POINT ( 'NONE',  ( 8.600005876649037262, -50.00000000000000000, -0.2541998246239300374 ) ) ;
#2056=CARTESIAN_POINT ( 'NONE',  ( -11.03470001049236160, -47.20000000000001705, 2.958453039083849045 ) ) ;
#2068=CARTESIAN_POINT ( 'NONE',  ( -8.599999999999996092, -50.00000000000000000, -1.093333333333363022 ) ) ;
#2077=CARTESIAN_POINT ( 'NONE',  ( -11.37702123033536061, -47.20000000000001705, 0.7471912688805021352 ) ) ;
#2085=CARTESIAN_POINT ( 'NONE',  ( 4.331939449206418935, -50.00000000000000000, 7.514224851275112194 ) ) ;
#2094=CARTESIAN_POINT ( 'NONE',  ( 5.285102517541700351, -47.20000000000001705, 6.877134118846478295 ) ) ;
#2097=CARTESIAN_POINT ( 'NONE',  ( -8.160064090060583197, -50.00000000000000000, 2.773119917861301964 ) ) ;
#2100=CARTESIAN_POINT ( 'NONE',  ( -8.489369361306263073, -50.00000000000000000, 1.403517616197273554 ) ) ;
#2104=DIRECTION ( 'NONE',  ( 1.000000000000000000, 0.000000000000000000, 0.000000000000000000 ) ) ;
#2112=CARTESIAN_POINT ( 'NONE',  ( 11.39999532361432522, -47.20000000000001705, 0.1755699507458462760 ) ) ;
#2131=CARTESIAN_POINT ( 'NONE',  ( 7.005833569765714586, -50.00000000000000000, 9.116201041261451365 ) ) ;
#2139=CARTESIAN_POINT ( 'NONE',  ( 8.599999999999996092, -50.00000000000000000, -1.366666666666861873 ) ) ;
#2142=CARTESIAN_POINT ( 'NONE',  ( -11.39539595717866405, -50.00000000000000000, 0.3739757293043588504 ) ) ;
#2143=CARTESIAN_POINT ( 'NONE',  ( -11.39999999999999680, -50.00000000000000000, -0.5466666666666361030 ) ) ;
#2145=CARTESIAN_POINT ( 'NONE',  ( 1.492255338562904043, -50.00000000000000000, 11.39999999999999680 ) ) ;
#2157=FILL_AREA_STYLE ('',( #620 ) ) ;
#2158=CARTESIAN_POINT ( 'NONE',  ( -2.982843918280285944, -50.00000000000000000, 11.10373667793902541 ) ) ;
#2161=AXIS2_PLACEMENT_3D ( 'NONE', #798, #3040, #1835 ) ;
#2162=CARTESIAN_POINT ( 'NONE',  ( -9.116201041287103735, -52.79999999999999716, 7.005833569791151128 ) ) ;
#2164=CARTESIAN_POINT ( 'NONE',  ( -9.198767304811452661, -48.81800434884508633, 0.7702149575309138463 ) ) ;
#2169=CARTESIAN_POINT ( 'NONE',  ( -8.530791689320901483, -50.00000000000000000, 1.124695299888049504 ) ) ;
#2173=EDGE_CURVE ( 'NONE', #403, #661, #1714, .T. ) ;
#2176=CARTESIAN_POINT ( 'NONE',  ( 11.40000778997679198, -47.20000000000001705, -0.2924664341912773247 ) ) ;
#2179=COLOUR_RGB ( '',0.8941176470588234615, 0.8941176470588234615, 0.8941176470588234615 ) ;
#2181=CARTESIAN_POINT ( 'NONE',  ( 10.81682914263883610, -50.00000000000000000, 3.675996170187548540 ) ) ;
#2187=CARTESIAN_POINT ( 'NONE',  ( -8.599999999999996092, -50.00000000000000000, -0.5466666666666361030 ) ) ;
#2189=CARTESIAN_POINT ( 'NONE',  ( 10.62090117298859226, -51.26516722440714346, -0.6209000891238516395 ) ) ;
#2191=CARTESIAN_POINT ( 'NONE',  ( 11.25335008359258282, -47.20000000000001705, 1.860476840074028360 ) ) ;
#2193=CARTESIAN_POINT ( 'NONE',  ( -10.76674801461903286, -51.18483196047731809, -0.7667480146190315260 ) ) ;
#2194=CARTESIAN_POINT ( 'NONE',  ( -5.742338339643776379, -52.79999999999999716, 9.960716663318299524 ) ) ;
#2196=CARTESIAN_POINT ( 'NONE',  ( 8.599999999999996092, -50.00000000000000000, -1.366666666666861873 ) ) ;
#2201=FACE_OUTER_BOUND ( 'NONE', #1293, .T. ) ;
#2205=CARTESIAN_POINT ( 'NONE',  ( 5.742338339644331491, -52.79999999999999716, 9.960716663318304853 ) ) ;
#2210=CARTESIAN_POINT ( 'NONE',  ( 11.30825875096042310, -52.79999999999999716, 1.490875164968454625 ) ) ;
#2214=CARTESIAN_POINT ( 'NONE',  ( 8.582665138674004268, -50.00000000000000000, 0.5636706063485154017 ) ) ;
#2216=CARTESIAN_POINT ( 'NONE',  ( 10.76729745289141604, -48.81576204415910780, -0.7672974528913893977 ) ) ;
#2219=CARTESIAN_POINT ( 'NONE',  ( -8.599996472200352571, -50.00000000000000000, 0.1525981975067654262 ) ) ;
#2223=CARTESIAN_POINT ( 'NONE',  ( -11.39999999999999680, -52.79999999999999716, -0.5466666666666361030 ) ) ;
#2228=CARTESIAN_POINT ( 'NONE',  ( 8.599996472200352571, -52.79999999999999716, 0.1525981975067867147 ) ) ;
#2230=CARTESIAN_POINT ( 'NONE',  ( 5.285102517541700351, -50.00000000000000000, 6.877134118846478295 ) ) ;
#2233=EDGE_CURVE ( 'NONE', #890, #365, #174, .T. ) ;
#2236=CARTESIAN_POINT ( 'NONE',  ( 8.324422814932070480, -50.00000000000000000, 2.231815450537910639 ) ) ;
#2240=CARTESIAN_POINT ( 'NONE',  ( -5.742338339643776379, -52.79999999999999716, 9.960716663318299524 ) ) ;
#2242=CARTESIAN_POINT ( 'NONE',  ( -10.00000000000001776, -51.39999999999999858, 1.734719586992576771E-19 ) ) ;
#2243=CARTESIAN_POINT ( 'NONE',  ( 1.125736483477000061, -52.79999999999999716, 8.599999999999996092 ) ) ;
#2245=CARTESIAN_POINT ( 'NONE',  ( -8.489369361306263073, -47.20000000000001705, 1.403517616197273554 ) ) ;
#2249=CARTESIAN_POINT ( 'NONE',  ( -8.599996472200352571, -47.20000000000001705, 0.1525981975067654817 ) ) ;
#2253=CARTESIAN_POINT ( 'NONE',  ( -11.39999532361432522, -52.79999999999999716, 0.1755699507458657049 ) ) ;
#2257=CARTESIAN_POINT ( 'NONE',  ( 10.81682914263855544, -52.79999999999999716, 3.675996170187548540 ) ) ;
#2259=CARTESIAN_POINT ( 'NONE',  ( 4.331939449206418047, -47.20000000000001705, 7.514224851275111305 ) ) ;
#2267=CARTESIAN_POINT ( 'NONE',  ( 11.40000778997679198, -52.79999999999999716, -0.2924664341912773247 ) ) ;
#2270=B_SPLINE_CURVE_WITH_KNOTS ( 'NONE', 3,
 ( #948, #724, #186, #1183, #1482, #2479, #1695, #2216, #1947, #3002, #474, #202 ),
 .UNSPECIFIED., .F., .F.,
 ( 4, 2, 2, 2, 2, 4 ),
 ( 0.002664946375549228936, 0.002999773306175310215, 0.003334600236801391060, 0.004004254098053570965, 0.004673907959305750003, 0.005343561820557929040 ),
 .UNSPECIFIED. ) ;
#2271=CARTESIAN_POINT ( 'NONE',  ( 8.160064090060387798, -50.00000000000000000, 2.773119917860402239 ) ) ;
#2278=( GEOMETRIC_REPRESENTATION_CONTEXT ( 3 ) GLOBAL_UNCERTAINTY_ASSIGNED_CONTEXT ( ( #2032 ) ) GLOBAL_UNIT_ASSIGNED_CONTEXT ( ( #382, #1904, #1390 ) ) REPRESENTATION_CONTEXT ( 'NONE', 'WORKASPACE' ) );
#2285=CARTESIAN_POINT ( 'NONE',  ( 8.906419880262733457, -50.95872650893685574, 1.034857390322859061 ) ) ;
#2286=CARTESIAN_POINT ( 'NONE',  ( 8.572276570257084671, -50.00000000000000000, 0.7042094815225934390 ) ) ;
#2291=CYLINDRICAL_SURFACE ( 'NONE', #2161, 1.399999999999999911 ) ;
#2301=CARTESIAN_POINT ( 'NONE',  ( 5.285102517541700351, -52.79999999999999716, 6.877134118846478295 ) ) ;
#2303=CARTESIAN_POINT ( 'NONE',  ( -8.489369361306263073, -50.00000000000000000, 1.403517616197273554 ) ) ;
#2308=CARTESIAN_POINT ( 'NONE',  ( 8.596526774713710850, -47.20000000000001705, 0.2821220414049827041 ) ) ;
#2310=ORIENTED_EDGE ( 'NONE', *, *, #306, .F. ) ;
#2317=CARTESIAN_POINT ( 'NONE',  ( 8.596526774713712626, -50.00000000000000000, 0.2821220414049827596 ) ) ;
#2319=CARTESIAN_POINT ( 'NONE',  ( 8.599999999999996092, -50.00000000000000000, -1.093333333333372126 ) ) ;
#2324=CARTESIAN_POINT ( 'NONE',  ( 2.982843918280841500, -47.20000000000001705, 11.10373667793903074 ) ) ;
#2334=CARTESIAN_POINT ( 'NONE',  ( 1.125736483477000061, -52.79999999999999716, 8.599999999999996092 ) ) ;
#2338=CARTESIAN_POINT ( 'NONE',  ( 8.582665138674004268, -50.00000000000000000, 0.5636706063485154017 ) ) ;
#2342=CARTESIAN_POINT ( 'NONE',  ( -7.513445500749801553, -47.20000000000001705, 4.333070140105379942 ) ) ;
#2349=CARTESIAN_POINT ( 'NONE',  ( -8.596526774713707297, -50.00000000000000000, 0.2821220414048196679 ) ) ;
#2358=CARTESIAN_POINT ( 'NONE',  ( -7.005833569763921354, -47.20000000000001705, 9.116201041262108618 ) ) ;
#2362=CARTESIAN_POINT ( 'NONE',  ( -8.485280282859317680, -50.00000000000000000, 1.400000000000003020 ) ) ;
#2377=CARTESIAN_POINT ( 'NONE',  ( -11.25335008359228794, -50.00000000000000000, 1.860476840075229621 ) ) ;
#2378=VERTEX_POINT ( 'NONE', #2445 ) ;
#2379=CARTESIAN_POINT ( 'NONE',  ( -8.485280282859317680, -50.00000000000000000, 1.400000000000003020 ) ) ;
#2393=CARTESIAN_POINT ( 'NONE',  ( -11.39999999999999680, -50.00000000000000000, -1.093333333333363022 ) ) ;
#2396=CARTESIAN_POINT ( 'NONE',  ( 11.39999999999999680, -47.20000000000001705, -1.366666666666861873 ) ) ;
#2406=SURFACE_STYLE_USAGE ( .BOTH. , #1406 ) ;
#2407=CARTESIAN_POINT ( 'NONE',  ( -11.39999999999999680, -47.20000000000001705, -0.5466666666666361030 ) ) ;
#2410=EDGE_CURVE ( 'NONE', #1696, #1290, #2270, .T. ) ;
#2411=CARTESIAN_POINT ( 'NONE',  ( 11.39999999999999680, -50.00000000000000000, -1.093333333333372126 ) ) ;
#2418=CARTESIAN_POINT ( 'NONE',  ( -8.599999999999996092, -50.00000000000000000, -1.093333333333363022 ) ) ;
#2423=CARTESIAN_POINT ( 'NONE',  ( 8.599999999999996092, -47.20000000000001705, -1.366666666666861873 ) ) ;
#2426=CARTESIAN_POINT ( 'NONE',  ( -10.81682914263834405, -50.00000000000000000, 3.675996170188739143 ) ) ;
#2432=CARTESIAN_POINT ( 'NONE',  ( 8.599999999999996092, -50.00000000000000000, -1.366666666666861873 ) ) ;
#2433=CARTESIAN_POINT ( 'NONE',  ( 8.767617449782822092, -49.18583174968845384, 1.157007882117269792 ) ) ;
#2437=STYLED_ITEM ( 'NONE', ( #1867 ), #1401 ) ;
#2438=CARTESIAN_POINT ( 'NONE',  ( 10.81682914263912210, -47.20000000000001705, 3.675996170187548540 ) ) ;
#2440=CARTESIAN_POINT ( 'NONE',  ( -8.768448914935611072, -50.81504429929021427, 1.156277961913375618 ) ) ;
#2441=CARTESIAN_POINT ( 'NONE',  ( -1.125736483477000061, -52.79999999999999716, 8.599999999999996092 ) ) ;
#2443=CARTESIAN_POINT ( 'NONE',  ( -8.160064090060583197, -47.20000000000001705, 2.773119917861301520 ) ) ;
#2444=B_SPLINE_CURVE_WITH_KNOTS ( 'NONE', 3,
 ( #2242, #1426, #704, #3233, #974, #687, #1959, #3248, #2440, #1992, #2996, #2750, #1704, #1670 ),
 .UNSPECIFIED., .F., .F.,
 ( 4, 2, 2, 2, 2, 2, 4 ),
 ( -7.483321517452871261E-06, 0.0003315069634277711215, 0.0006704972483729951726, 0.001348477818263447937, 0.002026458388153901027, 0.002365448673099125945, 0.002704438958044351297 ),
 .UNSPECIFIED. ) ;
#2445=CARTESIAN_POINT ( 'NONE',  ( -10.00000000000001776, -51.39999999999999858, 1.734719586992576771E-19 ) ) ;
#2449=CARTESIAN_POINT ( 'NONE',  ( 4.331939449206418935, -50.00000000000000000, 7.514224851275112194 ) ) ;
#2453=CARTESIAN_POINT ( 'NONE',  ( 8.600005876649037262, -47.20000000000001705, -0.2541998246239300374 ) ) ;
#2456=CARTESIAN_POINT ( 'NONE',  ( -8.599996472200352571, -52.79999999999999716, 0.1525981975067654817 ) ) ;
#2458=CARTESIAN_POINT ( 'NONE',  ( -5.285102517542626721, -50.00000000000000000, 6.877134118847252786 ) ) ;
#2462=CARTESIAN_POINT ( 'NONE',  ( 8.160064090060387798, -50.00000000000000000, 2.773119917860402239 ) ) ;
#2464=CARTESIAN_POINT ( 'NONE',  ( 11.33527052789730050, -50.43454227690138225, -1.335270527897303827 ) ) ;
#2468=CARTESIAN_POINT ( 'NONE',  ( 1.492255338562904265, -52.79999999999999716, 11.39999999999999680 ) ) ;
#2470=MECHANICAL_DESIGN_GEOMETRIC_PRESENTATION_REPRESENTATION('',(#1622),#460);
#2474=CARTESIAN_POINT ( 'NONE',  ( 8.596526774713710850, -52.79999999999999716, 0.2821220414049827041 ) ) ;
#2477=CARTESIAN_POINT ( 'NONE',  ( -8.596526774713705521, -47.20000000000001705, 0.2821220414048196123 ) ) ;
#2479=CARTESIAN_POINT ( 'NONE',  ( 11.16040725319407123, -49.19031162998081896, -1.160407253194085220 ) ) ;
#2482=CARTESIAN_POINT ( 'NONE',  ( -1.125736483476999839, -50.00000000000000000, 8.599999999999996092 ) ) ;
#2487=CARTESIAN_POINT ( 'NONE',  ( -11.36325033731753287, -52.79999999999999716, 0.9334869871344718684 ) ) ;
#2489=CARTESIAN_POINT ( 'NONE',  ( 11.39999999999999680, -50.00000000000000000, -1.400000000003877254 ) ) ;
#2490=CARTESIAN_POINT ( 'NONE',  ( -10.15747651436539734, -51.39999999999999858, -0.1574726269690627789 ) ) ;
#2492=CARTESIAN_POINT ( 'NONE',  ( 11.39999999999999680, -52.79999999999999716, -0.5466666666666269991 ) ) ;
#2495=CARTESIAN_POINT ( 'NONE',  ( -8.160064090060583197, -50.00000000000000000, 2.773119917861301964 ) ) ;
#2498=CARTESIAN_POINT ( 'NONE',  ( -11.39999999999999680, -47.20000000000001705, -0.5466666666666361030 ) ) ;
#2502=CARTESIAN_POINT ( 'NONE',  ( 11.39999999999999680, -50.00000000000000000, -0.5466666666666269991 ) ) ;
#2504=CARTESIAN_POINT ( 'NONE',  ( 9.116201041288118034, -52.79999999999999716, 7.005833569791843907 ) ) ;
#2506=CARTESIAN_POINT ( 'NONE',  ( -8.530791689320901483, -47.20000000000001705, 1.124695299888049504 ) ) ;
#2516=CARTESIAN_POINT ( 'NONE',  ( 11.39999999999999680, -50.00000000000000000, -1.639999999999997460 ) ) ;
#2519=CARTESIAN_POINT ( 'NONE',  ( -8.160064090060583197, -50.00000000000000000, 2.773119917861301964 ) ) ;
#2526=CARTESIAN_POINT ( 'NONE',  ( -10.31385090661583526, -48.62614420630684009, -0.3138474430211326549 ) ) ;
#2529=CARTESIAN_POINT ( 'NONE',  ( -8.599996472200352571, -52.79999999999999716, 0.1525981975067654817 ) ) ;
#2536=PRODUCT_DEFINITION ( 'UNKNOWN', '', #594, #40 ) ;
#2537=CARTESIAN_POINT ( 'NONE',  ( 4.331939449206418935, -50.00000000000000000, 7.514224851275112194 ) ) ;
#2548=CARTESIAN_POINT ( 'NONE',  ( 8.599996472200352571, -52.79999999999999716, 0.1525981975067867147 ) ) ;
#2554=CARTESIAN_POINT ( 'NONE',  ( -10.81682914263834405, -47.20000000000001705, 3.675996170188739143 ) ) ;
#2559=CARTESIAN_POINT ( 'NONE',  ( 9.677496024927361162, -51.36581032562466476, 0.3176491571778780054 ) ) ;
#2560=CARTESIAN_POINT ( 'NONE',  ( 6.877134118866902845, -50.00000000000000000, 5.285102517562147995 ) ) ;
#2564=CARTESIAN_POINT ( 'NONE',  ( -8.324422814933019055, -50.00000000000000000, 2.231815450536601464 ) ) ;
#2567=CARTESIAN_POINT ( 'NONE',  ( 5.742338339643197287, -47.20000000000001705, 9.960716663318304853 ) ) ;
#2577=CARTESIAN_POINT ( 'NONE',  ( -11.39999999999999680, -50.00000000000000000, -1.400000000000000133 ) ) ;
#2578=CARTESIAN_POINT ( 'NONE',  ( 2.250215587473118450, -52.79999999999999716, 8.376503107919017310 ) ) ;
#2582=CARTESIAN_POINT ( 'NONE',  ( 8.530791689320604831, -50.00000000000000000, 1.124695299888175182 ) ) ;
#2589=CARTESIAN_POINT ( 'NONE',  ( -8.599999999999996092, -47.20000000000001705, -0.5466666666666361030 ) ) ;
#2599=CARTESIAN_POINT ( 'NONE',  ( -8.599999999999996092, -50.00000000000000000, -1.366666666666159768 ) ) ;
#2610=CARTESIAN_POINT ( 'NONE',  ( 8.599999999999996092, -47.20000000000001705, -1.639999999999997460 ) ) ;
#2619=CARTESIAN_POINT ( 'NONE',  ( -6.877134118866000456, -50.00000000000000000, 5.285102517561346858 ) ) ;
#2622=( LENGTH_UNIT ( ) NAMED_UNIT ( * ) SI_UNIT ( .MILLI., .METRE. ) );
#2628=CARTESIAN_POINT ( 'NONE',  ( -9.959683570761574956, -50.00000000000000000, 5.743837162464267898 ) ) ;
#2636=ORIENTED_EDGE ( 'NONE', *, *, #697, .F. ) ;
#2639=CARTESIAN_POINT ( 'NONE',  ( -11.30825875096015665, -47.20000000000001705, 1.490875164968288979 ) ) ;
#2642=CARTESIAN_POINT ( 'NONE',  ( -11.36325033731753287, -52.79999999999999716, 0.9334869871344718684 ) ) ;
#2654=CARTESIAN_POINT ( 'NONE',  ( -11.39999999999999680, -50.00000000000000000, -1.639999999999997460 ) ) ;
#2655=CARTESIAN_POINT ( 'NONE',  ( -11.30825875096001454, -50.00000000000000000, 1.490875164968288757 ) ) ;
#2658=CARTESIAN_POINT ( 'NONE',  ( -11.25335008359243005, -52.79999999999999716, 1.860476840075229843 ) ) ;
#2662=CARTESIAN_POINT ( 'NONE',  ( -7.513445500749800665, -50.00000000000000000, 4.333070140105378165 ) ) ;
#2668=CARTESIAN_POINT ( 'NONE',  ( -11.39999999999999680, -47.20000000000001705, -1.093333333333363022 ) ) ;
#2669=CARTESIAN_POINT ( 'NONE',  ( -9.959683570761574956, -50.00000000000000000, 5.743837162464267898 ) ) ;
#2672=CARTESIAN_POINT ( 'NONE',  ( 11.39999999999999680, -47.20000000000001705, -0.5466666666666269991 ) ) ;
#2674=CARTESIAN_POINT ( 'NONE',  ( -9.595856219366988071, -48.65479562300421179, 0.3963015081148661412 ) ) ;
#2679=CARTESIAN_POINT ( 'NONE',  ( 8.599999999999996092, -50.00000000000000000, -0.5466666666666269991 ) ) ;
#2685=CARTESIAN_POINT ( 'NONE',  ( 11.39999999999999680, -47.20000000000001705, -1.639999999999997460 ) ) ;
#2689=CARTESIAN_POINT ( 'NONE',  ( -11.39999999999999680, -50.00000000000000000, -1.093333333333363022 ) ) ;
#2691=CARTESIAN_POINT ( 'NONE',  ( -8.599999999999996092, -47.20000000000001705, -1.093333333333363022 ) ) ;
#2700=CARTESIAN_POINT ( 'NONE',  ( -11.38641147205292192, -49.77694418854824221, -1.386411472052925697 ) ) ;
#2704=CARTESIAN_POINT ( 'NONE',  ( 5.742338339643197287, -47.20000000000001705, 9.960716663318304853 ) ) ;
#2707=CARTESIAN_POINT ( 'NONE',  ( 8.489369361306732031, -52.79999999999999716, 1.403517616196621409 ) ) ;
#2709=CARTESIAN_POINT ( 'NONE',  ( -8.599996472200352571, -50.00000000000000000, 0.1525981975067654262 ) ) ;
#2719=CARTESIAN_POINT ( 'NONE',  ( -2.982843918280285944, -52.79999999999999716, 11.10373667793902541 ) ) ;
#2722=CARTESIAN_POINT ( 'NONE',  ( 8.530791689320606608, -52.79999999999999716, 1.124695299888175182 ) ) ;
#2724=CARTESIAN_POINT ( 'NONE',  ( -8.599999999999996092, -47.20000000000001705, -1.639999999999997460 ) ) ;
#2728=CARTESIAN_POINT ( 'NONE',  ( -8.572276570256935457, -50.00000000000000000, 0.7042094815226510596 ) ) ;
#2733=CARTESIAN_POINT ( 'NONE',  ( 9.116201041287551377, -50.00000000000000000, 7.005833569791843018 ) ) ;
#2735=CARTESIAN_POINT ( 'NONE',  ( -10.31604092329497924, -51.37342103705936580, -0.3160374682705707761 ) ) ;
#2736=CARTESIAN_POINT ( 'NONE',  ( -8.530791689320901483, -52.79999999999999716, 1.124695299888049504 ) ) ;
#2739=CARTESIAN_POINT ( 'NONE',  ( -4.331939449206426929, -47.20000000000001705, 7.514224851276242845 ) ) ;
#2743=CARTESIAN_POINT ( 'NONE',  ( -2.250215587473127332, -47.20000000000001705, 8.376503107917878665 ) ) ;
#2746=CARTESIAN_POINT ( 'NONE',  ( -8.599999999999996092, -50.00000000000000000, -1.366666666666159768 ) ) ;
#2747=CARTESIAN_POINT ( 'NONE',  ( 11.39539595717845799, -52.79999999999999716, 0.3739757293042010877 ) ) ;
#2750=CARTESIAN_POINT ( 'NONE',  ( -8.502540660504315895, -50.22987518539498808, 1.385387373903827157 ) ) ;
#2751=CARTESIAN_POINT ( 'NONE',  ( -8.599999999999996092, -52.79999999999999716, -1.093333333333363022 ) ) ;
#2754=CARTESIAN_POINT ( 'NONE',  ( -8.596526774713707297, -50.00000000000000000, 0.2821220414048196679 ) ) ;
#2760=CARTESIAN_POINT ( 'NONE',  ( 11.36325033731732503, -50.00000000000000000, 0.9334869871343942638 ) ) ;
#2763=CARTESIAN_POINT ( 'NONE',  ( 11.36325033731725576, -52.79999999999999716, 0.9334869871343942638 ) ) ;
#2773=CARTESIAN_POINT ( 'NONE',  ( -8.599999999999996092, -52.79999999999999716, -0.5466666666666361030 ) ) ;
#2787=CARTESIAN_POINT ( 'NONE',  ( 8.160064090060387798, -52.79999999999999716, 2.773119917860402239 ) ) ;
#2793=CARTESIAN_POINT ( 'NONE',  ( 8.485280282859413603, -50.00000000000000000, 1.400000000000001021 ) ) ;
#2797=CARTESIAN_POINT ( 'NONE',  ( 8.600005876649037262, -47.20000000000001705, -0.2541998246239300374 ) ) ;
#2799=SHAPE_REPRESENTATION ( 'thread guide', ( #1692 ), #1379 ) ;
#2804=CARTESIAN_POINT ( 'NONE',  ( -8.324422814933019055, -50.00000000000000000, 2.231815450536601464 ) ) ;
#2808=CARTESIAN_POINT ( 'NONE',  ( 7.513445500750180805, -50.00000000000000000, 4.333070140107198043 ) ) ;
#2809=CARTESIAN_POINT ( 'NONE',  ( 8.160064090060387798, -50.00000000000000000, 2.773119917860402239 ) ) ;
#2812=CARTESIAN_POINT ( 'NONE',  ( -8.530791689320901483, -47.20000000000001705, 1.124695299888049504 ) ) ;
#2819=CARTESIAN_POINT ( 'NONE',  ( -4.331939449206426929, -52.79999999999999716, 7.514224851276242845 ) ) ;
#2823=CARTESIAN_POINT ( 'NONE',  ( -1.125736483476999839, -50.00000000000000000, 8.599999999999996092 ) ) ;
#2824=CARTESIAN_POINT ( 'NONE',  ( 8.485280282859413603, -50.00000000000000000, 1.400000000000001021 ) ) ;
#2829=CARTESIAN_POINT ( 'NONE',  ( -11.39999532361432522, -47.20000000000001705, 0.1755699507458657049 ) ) ;
#2837=CARTESIAN_POINT ( 'NONE',  ( 8.582665138674004268, -52.79999999999999716, 0.5636706063485154017 ) ) ;
#2844=ORIENTED_EDGE ( 'NONE', *, *, #15, .F. ) ;
#2847=CARTESIAN_POINT ( 'NONE',  ( -9.116201041289377471, -47.20000000000001705, 7.005833569791151128 ) ) ;
#2850=DIRECTION ( 'NONE',  ( -1.000000000000000000, -0.000000000000000000, -0.000000000000000000 ) ) ;
#2853=CARTESIAN_POINT ( 'NONE',  ( -7.513445500749800665, -50.00000000000000000, 4.333070140105378165 ) ) ;
#2858=CARTESIAN_POINT ( 'NONE',  ( 8.530791689320606608, -52.79999999999999716, 1.124695299888175182 ) ) ;
#2866=CARTESIAN_POINT ( 'NONE',  ( 9.959683570760574867, -50.00000000000000000, 5.743837162466680191 ) ) ;
#2867=CARTESIAN_POINT ( 'NONE',  ( -8.555056788725856620, -49.54949886534770087, 1.341113681525112122 ) ) ;
#2869=CARTESIAN_POINT ( 'NONE',  ( -8.469856736028225086, -50.00000000000000000, 1.493482969799723170 ) ) ;
#2872=LINE ( 'NONE', #1619, #93 ) ;
#2873=B_SPLINE_CURVE_WITH_KNOTS ( 'NONE', 3,
 ( #2965, #2490, #2735, #1443, #2193, #149, #1226, #2945, #3212, #926, #1737, #452, #212, #1940 ),
 .UNSPECIFIED., .F., .F.,
 ( 4, 2, 2, 2, 2, 2, 4 ),
 ( -7.483321455836769026E-06, 0.0006606241027954191589, 0.001328731527046675062, 0.001662785239172306700, 0.001996838951297938338, 0.002330892663423569759, 0.002664946375549201180 ),
 .UNSPECIFIED. ) ;
#2878=CARTESIAN_POINT ( 'NONE',  ( -11.39999999999999680, -47.20000000000001705, -1.366666666666159546 ) ) ;
#2882=CARTESIAN_POINT ( 'NONE',  ( -11.39999999999999680, -52.79999999999999716, -0.5466666666666361030 ) ) ;
#2887=ORIENTED_EDGE ( 'NONE', *, *, #1442, .F. ) ;
#2891=ORIENTED_EDGE ( 'NONE', *, *, #889, .T. ) ;
#2894=( NAMED_UNIT ( * ) PLANE_ANGLE_UNIT ( ) SI_UNIT ( $, .RADIAN. ) );
#2895=CARTESIAN_POINT ( 'NONE',  ( -11.39999532361432522, -50.00000000000000000, 0.1755699507458657049 ) ) ;
#2898=CARTESIAN_POINT ( 'NONE',  ( 11.36325033731739609, -47.20000000000001705, 0.9334869871343942638 ) ) ;
#2907=CARTESIAN_POINT ( 'NONE',  ( -8.599999999999996092, -50.00000000000000000, -1.639999999999997460 ) ) ;
#2908=CARTESIAN_POINT ( 'NONE',  ( 9.198767304811504175, -48.81800434884510764, 0.7702149575309279461 ) ) ;
#2913=CARTESIAN_POINT ( 'NONE',  ( 1.492255338562904265, -47.20000000000001705, 11.39999999999999680 ) ) ;
#2914=CARTESIAN_POINT ( 'NONE',  ( -11.03470001049207916, -50.00000000000000000, 2.958453039083848601 ) ) ;
#2916=CARTESIAN_POINT ( 'NONE',  ( -11.39999532361432522, -50.00000000000000000, 0.1755699507458657049 ) ) ;
#2926=CARTESIAN_POINT ( 'NONE',  ( -11.03470001049207916, -50.00000000000000000, 2.958453039083848601 ) ) ;
#2930=CARTESIAN_POINT ( 'NONE',  ( 11.39999999999999680, -47.20000000000001705, -1.093333333333372126 ) ) ;
#2932=CARTESIAN_POINT ( 'NONE',  ( 8.530791689320606608, -47.20000000000001705, 1.124695299888175182 ) ) ;
#2938=CARTESIAN_POINT ( 'NONE',  ( -8.324422814933019055, -50.00000000000000000, 2.231815450536601464 ) ) ;
#2939=CARTESIAN_POINT ( 'NONE',  ( 8.555056788725931227, -49.54949886534768666, 1.341113681525113455 ) ) ;
#2943=CARTESIAN_POINT ( 'NONE',  ( 8.599999999999996092, -47.20000000000001705, -1.639999999999997460 ) ) ;
#2944=CARTESIAN_POINT ( 'NONE',  ( -5.742338339643776379, -50.00000000000000000, 9.960716663318299524 ) ) ;
#2945=CARTESIAN_POINT ( 'NONE',  ( -11.15228598338264909, -50.80068377669682178, -1.152285983382659751 ) ) ;
#2949=CARTESIAN_POINT ( 'NONE',  ( 8.160064090060387798, -52.79999999999999716, 2.773119917860402239 ) ) ;
#2951=CARTESIAN_POINT ( 'NONE',  ( 8.599999999999996092, -50.00000000000000000, -1.093333333333372126 ) ) ;
#2958=CARTESIAN_POINT ( 'NONE',  ( -8.160064090060583197, -50.00000000000000000, 2.773119917861301964 ) ) ;
#2963=CARTESIAN_POINT ( 'NONE',  ( -11.25335008359243005, -52.79999999999999716, 1.860476840075229843 ) ) ;
#2965=CARTESIAN_POINT ( 'NONE',  ( -10.00000000000001776, -51.39999999999999858, 1.734719586992576771E-19 ) ) ;
#2966=B_SPLINE_CURVE_WITH_KNOTS ( 'NONE', 3,
 ( #2362, #2869, #1081, #1332, #2097, #2853, #1599, #341, #1348, #91, #1100, #3124, #1366, #2537, #1324, #3096, #83, #2809, #1092, #1340, #1818, #2793 ),
 .UNSPECIFIED., .F., .F.,
 ( 4, 2, 2, 2, 2, 2, 2, 2, 2, 2, 4 ),
 ( 0.05198376726129744912, 0.06250000000000000000, 0.1250000000000000000, 0.2500000000000000000, 0.3750000000000000000, 0.5000000000000000000, 0.6250000000000000000, 0.7500000000000000000, 0.8750000000000000000, 0.9375000000000000000, 0.9480162327386928434 ),
 .UNSPECIFIED. ) ;
#2967=CARTESIAN_POINT ( 'NONE',  ( 7.513445500750181694, -52.79999999999999716, 4.333070140107198043 ) ) ;
#2968=ORIENTED_EDGE ( 'NONE', *, *, #507, .T. ) ;
#2969=CARTESIAN_POINT ( 'NONE',  ( -8.599999999999996092, -47.20000000000001705, -0.5466666666666361030 ) ) ;
#2974=CARTESIAN_POINT ( 'NONE',  ( -8.596526774713707297, -50.00000000000000000, 0.2821220414048196679 ) ) ;
#2978=CARTESIAN_POINT ( 'NONE',  ( -11.39999999999999680, -52.79999999999999716, -1.366666666666159546 ) ) ;
#2979=CARTESIAN_POINT ( 'NONE',  ( 9.116201041287551377, -50.00000000000000000, 7.005833569791843018 ) ) ;
#2981=CARTESIAN_POINT ( 'NONE',  ( 8.599999999999996092, -52.79999999999999716, -1.093333333333372126 ) ) ;
#2983=CARTESIAN_POINT ( 'NONE',  ( 8.599996472200352571, -50.00000000000000000, 0.1525981975067866592 ) ) ;
#2989=CARTESIAN_POINT ( 'NONE',  ( -5.742338339643776379, -47.20000000000001705, 9.960716663318299524 ) ) ;
#2992=CARTESIAN_POINT ( 'NONE',  ( -8.599999999999996092, -50.00000000000000000, -1.093333333333363022 ) ) ;
#2993=CARTESIAN_POINT ( 'NONE',  ( -11.39999999999999680, -52.79999999999999716, -1.639999999999997460 ) ) ;
#2994=CARTESIAN_POINT ( 'NONE',  ( 11.30825875096028099, -50.00000000000000000, 1.490875164968454181 ) ) ;
#2996=CARTESIAN_POINT ( 'NONE',  ( -8.564669657330886920, -50.44377267524131270, 1.332368788789987768 ) ) ;
#2998=CARTESIAN_POINT ( 'NONE',  ( -8.599999999999996092, -50.00000000000000000, -1.093333333333363022 ) ) ;
#3001=CARTESIAN_POINT ( 'NONE',  ( 6.877134118866901957, -47.20000000000001705, 5.285102517562147995 ) ) ;
#3002=CARTESIAN_POINT ( 'NONE',  ( 10.31385090661579795, -48.62614420630679746, -0.3138474430211479760 ) ) ;
#3004=CARTESIAN_POINT ( 'NONE',  ( -6.877134118866001344, -47.20000000000001705, 5.285102517561345969 ) ) ;
#3005=CARTESIAN_POINT ( 'NONE',  ( -10.76729745289139473, -48.81576204415910070, -0.7672974528914079384 ) ) ;
#3008=CARTESIAN_POINT ( 'NONE',  ( 8.485280282859415379, -50.11569792258605816, 1.400000000000001243 ) ) ;
#3009=CARTESIAN_POINT ( 'NONE',  ( 11.39999999999999680, -52.79999999999999716, -1.366666666666861873 ) ) ;
#3012=( NAMED_UNIT ( * ) SI_UNIT ( $, .STERADIAN. ) SOLID_ANGLE_UNIT ( ) );
#3013=CARTESIAN_POINT ( 'NONE',  ( -7.513445500749801553, -52.79999999999999716, 4.333070140105379942 ) ) ;
#3020=DIRECTION ( 'NONE',  ( -1.000000000000000000, -0.000000000000000000, -0.000000000000000000 ) ) ;
#3023=CARTESIAN_POINT ( 'NONE',  ( 11.39999532361432522, -50.00000000000000000, 0.1755699507458462760 ) ) ;
#3025=EDGE_CURVE ( 'NONE', #661, #365, #3055, .T. ) ;
#3026=CARTESIAN_POINT ( 'NONE',  ( 8.599999999999996092, -50.00000000000000000, -1.366666666666861873 ) ) ;
#3035=CARTESIAN_POINT ( 'NONE',  ( -5.285102517542626721, -52.79999999999999716, 6.877134118847253674 ) ) ;
#3040=DIRECTION ( 'NONE',  ( -1.000000000000000000, -0.000000000000000000, -0.000000000000000000 ) ) ;
#3053=CARTESIAN_POINT ( 'NONE',  ( 7.513445500750181694, -52.79999999999999716, 4.333070140107198043 ) ) ;
#3055=B_SPLINE_CURVE_WITH_KNOTS ( 'NONE', 3,
 ( #2379, #1099, #2867, #137, #1660, #2164, #629, #2674, #3172, #660, #610, #1615 ),
 .UNSPECIFIED., .F., .F.,
 ( 4, 2, 2, 2, 2, 4 ),
 ( 0.002704438958044351297, 0.003382491784598461778, 0.004060544611152572259, 0.004738597437706682305, 0.005077623850983738196, 0.005416650264260793220 ),
 .UNSPECIFIED. ) ;
#3065=CARTESIAN_POINT ( 'NONE',  ( -1.492255338562904265, -47.20000000000001705, 11.39999999999999680 ) ) ;
#3071=CARTESIAN_POINT ( 'NONE',  ( -8.485280282859317680, -50.00000000000000000, 1.400000000000003020 ) ) ;
#3072=CARTESIAN_POINT ( 'NONE',  ( 8.599999999999996092, -52.79999999999999716, -1.366666666666861873 ) ) ;
#3075=CARTESIAN_POINT ( 'NONE',  ( 0.000000000000000000, 0.000000000000000000, 0.000000000000000000 ) ) ;
#3078=ORIENTED_EDGE ( 'NONE', *, *, #889, .F. ) ;
#3081=CARTESIAN_POINT ( 'NONE',  ( 9.959683570760009985, -47.20000000000001705, 5.743837162466679302 ) ) ;
#3089=CARTESIAN_POINT ( 'NONE',  ( -8.582665138674013150, -52.79999999999999716, 0.5636706063486748297 ) ) ;
#3096=CARTESIAN_POINT ( 'NONE',  ( 6.877134118866902845, -50.00000000000000000, 5.285102517562147995 ) ) ;
#3100=ADVANCED_FACE ( 'NONE', ( #109 ), #1133, .T. ) ;
#3101=CARTESIAN_POINT ( 'NONE',  ( -11.39999999999999680, -47.20000000000001705, -1.366666666666159546 ) ) ;
#3109=CARTESIAN_POINT ( 'NONE',  ( -8.160064090060583197, -52.79999999999999716, 2.773119917861301520 ) ) ;
#3110=ORIENTED_EDGE ( 'NONE', *, *, #306, .T. ) ;
#3120=CARTESIAN_POINT ( 'NONE',  ( -11.03470001049207916, -50.00000000000000000, 2.958453039083848601 ) ) ;
#3124=CARTESIAN_POINT ( 'NONE',  ( 1.125736483476999839, -50.00000000000000000, 8.599999999999996092 ) ) ;
#3126=B_SPLINE_CURVE_WITH_KNOTS ( 'NONE', 3,
 ( #530, #1237, #481, #2559, #1554, #777, #292, #2285, #1491, #12, #274, #1282, #3008, #2048 ),
 .UNSPECIFIED., .F., .F.,
 ( 4, 2, 2, 2, 2, 2, 4 ),
 ( -7.483321517480581097E-06, 0.0003315069634265197353, 0.0006704972483705200475, 0.001348477818258529129, 0.002026458388146537993, 0.002365448673090551641, 0.002704438958034565722 ),
 .UNSPECIFIED. ) ;
#3133=CARTESIAN_POINT ( 'NONE',  ( 11.39999999999999680, -47.20000000000001705, -1.093333333333372126 ) ) ;
#3134=PRODUCT_DEFINITION_SHAPE ( 'NONE', 'NONE',  #2536 ) ;
#3135=CARTESIAN_POINT ( 'NONE',  ( -11.39999999999999680, -50.00000000000000711, -1.206666666667079335 ) ) ;
#3139=CARTESIAN_POINT ( 'NONE',  ( -11.37702123033528778, -50.00000000000000000, 0.7471912688805022462 ) ) ;
#3140=CARTESIAN_POINT ( 'NONE',  ( 11.64000000000000057, -50.00000000000000000, 0.000000000000000000 ) ) ;
#3149=CARTESIAN_POINT ( 'NONE',  ( -9.116201041288242379, -50.00000000000000000, 7.005833569791151128 ) ) ;
#3150=CARTESIAN_POINT ( 'NONE',  ( -11.39539595717866405, -50.00000000000000000, 0.3739757293043588504 ) ) ;
#3152=CARTESIAN_POINT ( 'NONE',  ( 5.742338339643763945, -50.00000000000000000, 9.960716663318306630 ) ) ;
#3166=CARTESIAN_POINT ( 'NONE',  ( 8.596526774713710850, -47.20000000000001705, 0.2821220414049827041 ) ) ;
#3167=CARTESIAN_POINT ( 'NONE',  ( -11.25335008359228794, -50.00000000000000000, 1.860476840075229621 ) ) ;
#3169=CARTESIAN_POINT ( 'NONE',  ( -11.39999999999999680, -52.79999999999999716, -1.366666666666159546 ) ) ;
#3172=CARTESIAN_POINT ( 'NONE',  ( -9.676554491074602637, -48.63437908886124461, 0.3185635799549239588 ) ) ;
#3178=CARTESIAN_POINT ( 'NONE',  ( -8.489369361306263073, -50.00000000000000000, 1.403517616197273554 ) ) ;
#3183=CARTESIAN_POINT ( 'NONE',  ( -11.39999999999999680, -47.20000000000001705, -1.639999999999997460 ) ) ;
#3185=CARTESIAN_POINT ( 'NONE',  ( 11.37702123033542279, -50.00000000000000000, 0.7471912688806704450 ) ) ;
#3193=CARTESIAN_POINT ( 'NONE',  ( 11.39999999999999503, -50.11112248448768014, -1.399999999999995470 ) ) ;
#3196=CARTESIAN_POINT ( 'NONE',  ( -11.36325033731746004, -50.00000000000000000, 0.9334869871344717573 ) ) ;
#3197=CARTESIAN_POINT ( 'NONE',  ( -11.37702123033528778, -50.00000000000000000, 0.7471912688805022462 ) ) ;
#3199=CARTESIAN_POINT ( 'NONE',  ( -8.324422814933019055, -52.79999999999999716, 2.231815450536601020 ) ) ;
#3201=CARTESIAN_POINT ( 'NONE',  ( -8.530791689320901483, -50.00000000000000000, 1.124695299888049504 ) ) ;
#3210=CARTESIAN_POINT ( 'NONE',  ( -11.30825875095987421, -52.79999999999999716, 1.490875164968288757 ) ) ;
#3212=CARTESIAN_POINT ( 'NONE',  ( -11.20659079646780221, -50.71729705017419576, -1.206590796467802207 ) ) ;
#3213=CARTESIAN_POINT ( 'NONE',  ( -8.489369361306263073, -52.79999999999999716, 1.403517616197273554 ) ) ;
#3215=CARTESIAN_POINT ( 'NONE',  ( 8.600005876649037262, -50.00000000000000000, -0.2541998246239300374 ) ) ;
#3220=APPLICATION_CONTEXT ( 'automotive_design' ) ;
#3227=CARTESIAN_POINT ( 'NONE',  ( 10.15747651431146892, -51.40000000000001279, -0.1574726270229690750 ) ) ;
#3230=MECHANICAL_DESIGN_GEOMETRIC_PRESENTATION_REPRESENTATION('',(#2437),#2278);
#3231=CARTESIAN_POINT ( 'NONE',  ( 11.25335008359272493, -50.00000000000000000, 1.860476840074170246 ) ) ;
#3233=CARTESIAN_POINT ( 'NONE',  ( -9.677496024926982798, -51.36581032562460791, 0.3176491571783061074 ) ) ;
#3234=CARTESIAN_POINT ( 'NONE',  ( 11.25335008359286704, -52.79999999999999716, 1.860476840074311911 ) ) ;
#3236=CARTESIAN_POINT ( 'NONE',  ( -8.572276570256935457, -47.20000000000001705, 0.7042094815226510596 ) ) ;
#3246=CARTESIAN_POINT ( 'NONE',  ( 11.37702123033549384, -52.79999999999999716, 0.7471912688806703340 ) ) ;
#3248=CARTESIAN_POINT ( 'NONE',  ( -8.906419880262294697, -50.95872650893633704, 1.034857390323304926 ) ) ;
#3249=CARTESIAN_POINT ( 'NONE',  ( -8.599999999999996092, -50.00000000000000000, -1.639999999999997460 ) ) ;
#3251=CARTESIAN_POINT ( 'NONE',  ( 1.125736483477000061, -47.20000000000001705, 8.599999999999996092 ) ) ;
#3255=CARTESIAN_POINT ( 'NONE',  ( -1.125736483477000061, -47.20000000000001705, 8.599999999999996092 ) ) ;
#3257=CARTESIAN_POINT ( 'NONE',  ( 11.03475136337292639, -50.94770623811574950, -1.034751363372934829 ) ) ;
#3261=CARTESIAN_POINT ( 'NONE',  ( -9.116201041287103735, -52.79999999999999716, 7.005833569791151128 ) ) ;
#3262=CARTESIAN_POINT ( 'NONE',  ( 1.492255338562904043, -50.00000000000000000, 11.39999999999999680 ) ) ;
#3265=CARTESIAN_POINT ( 'NONE',  ( -8.600005876649037262, -52.79999999999999716, -0.2541998246238979520 ) ) ;
#3287=COLOUR_RGB('Light Blue',0.38,0.62,0.78);
#3288=FILL_AREA_STYLE_COLOUR('',#3287);
#3289=FILL_AREA_STYLE('',(#3288));
#3290=SURFACE_STYLE_FILL_AREA(#3289);
#3291=SURFACE_SIDE_STYLE('',(#3290));
#3292=SURFACE_STYLE_USAGE(.BOTH.,#3291);
#3293=PRESENTATION_STYLE_ASSIGNMENT((#3292));
ENDSEC;
END-ISO-10303-21;
